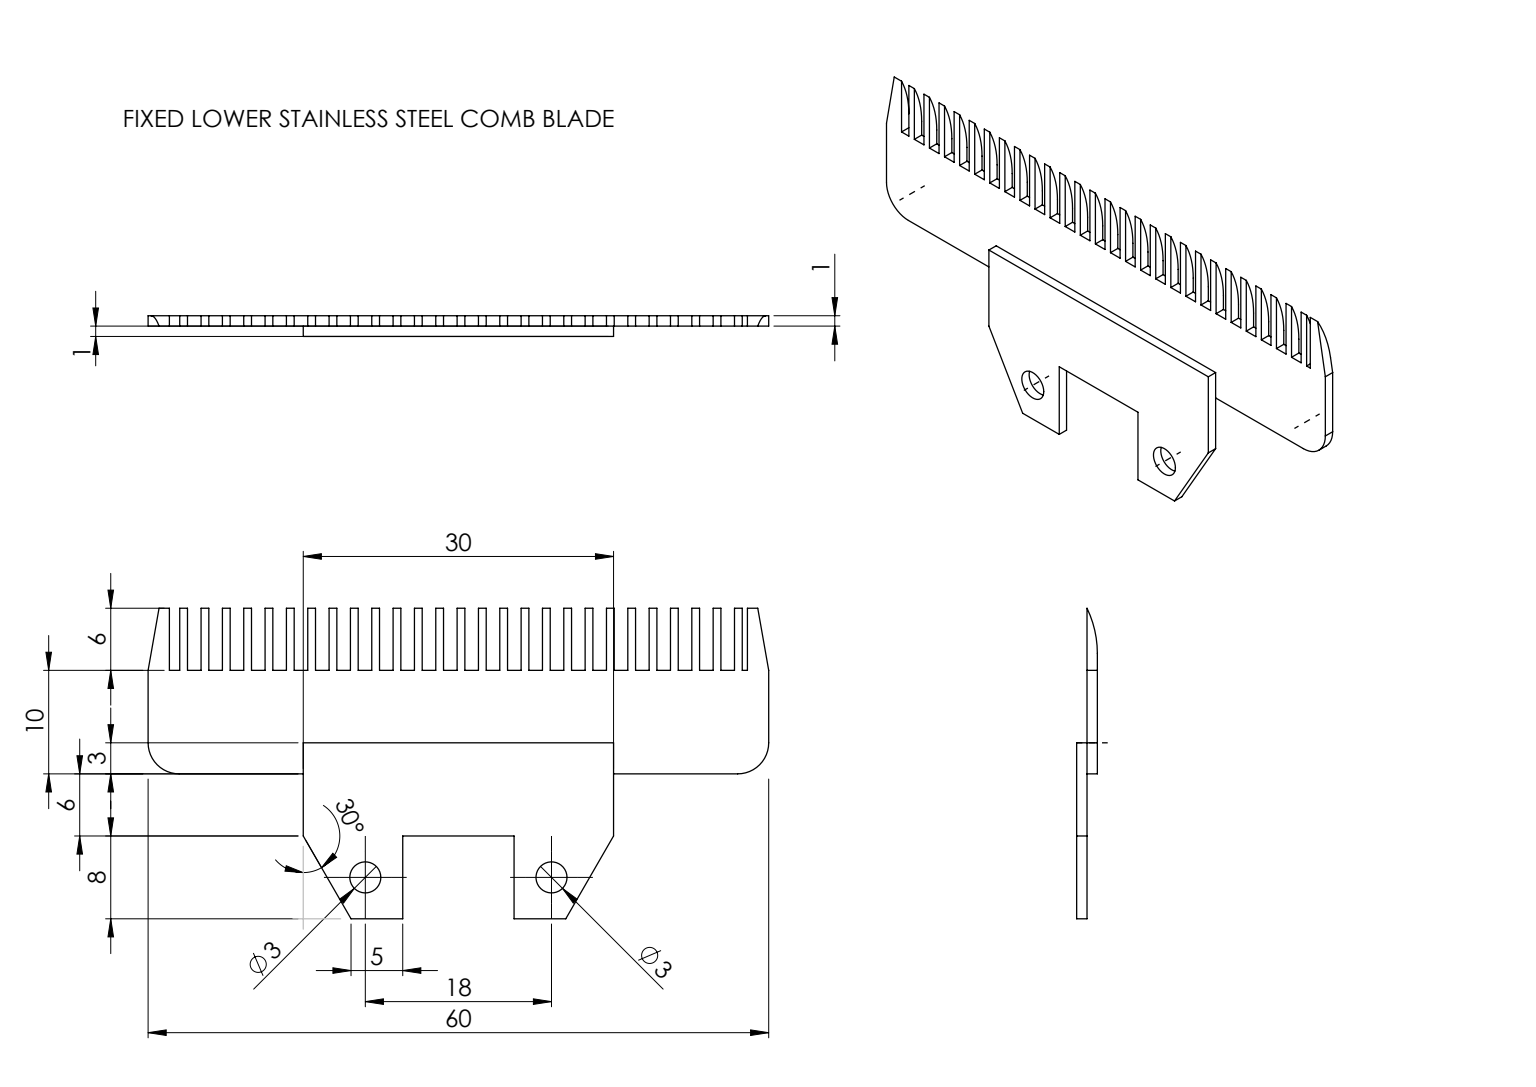
ISO-10303-21;
HEADER;
FILE_DESCRIPTION (('STEP AP214'),
    '1' );
FILE_NAME ('Fixed Lower Stainless Steel Comb Blade.step',
    '2026-10-04T16:38:04',
    ( '' ),
    ( '' ),
    'SwSTEP 2.0',
    'SolidWorks 2026',
    '' );
FILE_SCHEMA (( 'AUTOMOTIVE_DESIGN' ));
ENDSEC;

DATA;
#1=EDGE_CURVE ( 'NONE', #8973, #13899, #6324, .T. ) ;
#2=DIRECTION ( 'NONE',  ( -1.000000000000000000, 0.000000000000000000, 0.000000000000000000 ) ) ;
#6=AXIS2_PLACEMENT_3D ( 'NONE', #19220, #15754, #1437 ) ;
#8=CARTESIAN_POINT ( 'NONE',  ( -22.81633994409548549, 11.64110105645932691, 0.000000000000000000 ) ) ;
#13=VERTEX_POINT ( 'NONE', #12698 ) ;
#20=CARTESIAN_POINT ( 'NONE',  ( 29.44326362367961636, 13.15740888934567288, -2.785412301099487325E-16 ) ) ;
#23=CIRCLE ( 'NONE', #12706, 10.00000000000000000 ) ;
#24=DIRECTION ( 'NONE',  ( 1.000000000000000000, 0.000000000000000000, 0.000000000000000000 ) ) ;
#27=EDGE_CURVE ( 'NONE', #6657, #12771, #12900, .T. ) ;
#31=CARTESIAN_POINT ( 'NONE',  ( -18.69064177244175795, 11.64110105645932691, 0.000000000000000000 ) ) ;
#36=ADVANCED_FACE ( 'NONE', ( #7996 ), #7800, .T. ) ;
#38=CARTESIAN_POINT ( 'NONE',  ( 0.000000000000000000, 10.00000000000000000, 1.000000000000000000 ) ) ;
#39=CIRCLE ( 'NONE', #18741, 9.999999999999998224 ) ;
#43=VECTOR ( 'NONE', #1167, 1000.000000000000000 ) ;
#50=PLANE ( 'NONE',  #13438 ) ;
#51=PLANE ( 'NONE',  #17586 ) ;
#52=DIRECTION ( 'NONE',  ( 0.000000000000000000, 0.000000000000000000, 1.000000000000000000 ) ) ;
#62=DIRECTION ( 'NONE',  ( -5.782411586589356653E-16, 1.000000000000000000, 0.000000000000000000 ) ) ;
#73=AXIS2_PLACEMENT_3D ( 'NONE', #7626, #20402, #7929 ) ;
#74=DIRECTION ( 'NONE',  ( 1.000000000000000000, 0.000000000000000000, -0.000000000000000000 ) ) ;
#80=DIRECTION ( 'NONE',  ( -0.000000000000000000, -0.000000000000000000, -1.000000000000000000 ) ) ;
#81=EDGE_CURVE ( 'NONE', #12312, #20463, #4960, .T. ) ;
#93=DIRECTION ( 'NONE',  ( -0.000000000000000000, -0.000000000000000000, -1.000000000000000000 ) ) ;
#100=DIRECTION ( 'NONE',  ( 0.000000000000000000, 1.000000000000000000, 0.000000000000000000 ) ) ;
#104=ORIENTED_EDGE ( 'NONE', *, *, #13146, .F. ) ;
#118=EDGE_CURVE ( 'NONE', #8944, #9004, #361, .T. ) ;
#124=CARTESIAN_POINT ( 'NONE',  ( 27.94203811574920948, 16.00000000000000000, 1.000000000000000000 ) ) ;
#127=EDGE_LOOP ( 'NONE', ( #2197, #15477, #13303, #7881 ) ) ;
#129=CARTESIAN_POINT ( 'NONE',  ( 0.000000000000000000, 11.64110105645932691, 10.00000000000000000 ) ) ;
#130=FACE_OUTER_BOUND ( 'NONE', #18306, .T. ) ;
#131=APPLICATION_CONTEXT ( 'automotive_design' ) ;
#136=DIRECTION ( 'NONE',  ( 0.000000000000000000, 0.000000000000000000, -1.000000000000000000 ) ) ;
#140=ORIENTED_EDGE ( 'NONE', *, *, #2638, .T. ) ;
#142=CARTESIAN_POINT ( 'NONE',  ( 6.063547257480584207, 10.00000000000000000, 1.000000000000000000 ) ) ;
#145=EDGE_LOOP ( 'NONE', ( #572, #13357 ) ) ;
#149=EDGE_LOOP ( 'NONE', ( #17432, #19814, #17504, #3948 ) ) ;
#151=ORIENTED_EDGE ( 'NONE', *, *, #14900, .F. ) ;
#152=CARTESIAN_POINT ( 'NONE',  ( -27.94203811574921659, 9.999999999999998224, 1.000000000000000000 ) ) ;
#157=CARTESIAN_POINT ( 'NONE',  ( 0.000000000000000000, 10.00000000000000000, 1.000000000000000000 ) ) ;
#160=CARTESIAN_POINT ( 'NONE',  ( 27.00000000000000000, 3.000000000000000000, 1.000000000000000000 ) ) ;
#162=DIRECTION ( 'NONE',  ( -0.000000000000000000, -0.000000000000000000, -1.000000000000000000 ) ) ;
#171=ORIENTED_EDGE ( 'NONE', *, *, #6216, .T. ) ;
#172=ORIENTED_EDGE ( 'NONE', *, *, #1116, .F. ) ;
#173=DIRECTION ( 'NONE',  ( -0.000000000000000000, -0.000000000000000000, -1.000000000000000000 ) ) ;
#175=VERTEX_POINT ( 'NONE', #3806 ) ;
#176=CARTESIAN_POINT ( 'NONE',  ( -15.00000000000000000, 3.000000000000000000, 1.000000000000000000 ) ) ;
#184=EDGE_CURVE ( 'NONE', #2924, #1770, #13210, .T. ) ;
#193=VERTEX_POINT ( 'NONE', #561 ) ;
#194=FACE_OUTER_BOUND ( 'NONE', #14246, .T. ) ;
#196=LINE ( 'NONE', #13157, #16335 ) ;
#197=EDGE_CURVE ( 'NONE', #4053, #10774, #19608, .T. ) ;
#201=CARTESIAN_POINT ( 'NONE',  ( -8.376396343307449754, 11.64110105645932691, 0.000000000000000000 ) ) ;
#204=DIRECTION ( 'NONE',  ( 0.000000000000000000, -1.000000000000000000, 0.000000000000000000 ) ) ;
#219=CYLINDRICAL_SURFACE ( 'NONE', #18842, 10.00000000000000000 ) ;
#221=ORIENTED_EDGE ( 'NONE', *, *, #17663, .T. ) ;
#222=CARTESIAN_POINT ( 'NONE',  ( -14.56494360078803396, 0.000000000000000000, 0.000000000000000000 ) ) ;
#223=CYLINDRICAL_SURFACE ( 'NONE', #8699, 10.00000000000000000 ) ;
#226=CARTESIAN_POINT ( 'NONE',  ( 0.000000000000000000, 11.64110105645932691, 10.00000000000000000 ) ) ;
#227=EDGE_CURVE ( 'NONE', #2917, #11113, #5373, .T. ) ;
#234=EDGE_LOOP ( 'NONE', ( #6120, #13458, #16622, #14444 ) ) ;
#235=VECTOR ( 'NONE', #10575, 1000.000000000000000 ) ;
#240=EDGE_LOOP ( 'NONE', ( #2876, #19889, #3545, #20179 ) ) ;
#243=CARTESIAN_POINT ( 'NONE',  ( -0.000000000000000000, 10.00000000000000000, 0.000000000000000000 ) ) ;
#245=ORIENTED_EDGE ( 'NONE', *, *, #7610, .F. ) ;
#246=LINE ( 'NONE', #152, #17116 ) ;
#251=CARTESIAN_POINT ( 'NONE',  ( -7.500000000000000888, -9.999999999999992895, 1.000000000000000000 ) ) ;
#252=VECTOR ( 'NONE', #1364, 1000.000000000000000 ) ;
#256=LINE ( 'NONE', #3402, #19673 ) ;
#264=ADVANCED_FACE ( 'NONE', ( #16459 ), #18242, .T. ) ;
#269=CARTESIAN_POINT ( 'NONE',  ( -0.000000000000000000, 11.64110105645932691, 0.000000000000000000 ) ) ;
#271=ORIENTED_EDGE ( 'NONE', *, *, #10983, .T. ) ;
#273=VECTOR ( 'NONE', #18703, 1000.000000000000000 ) ;
#276=DIRECTION ( 'NONE',  ( 0.000000000000000000, 0.000000000000000000, 1.000000000000000000 ) ) ;
#280=AXIS2_PLACEMENT_3D ( 'NONE', #10758, #15558, #17129 ) ;
#283=FILL_AREA_STYLE ('',( #16193 ) ) ;
#285=DIRECTION ( 'NONE',  ( 1.000000000000000000, 0.000000000000000000, -0.000000000000000000 ) ) ;
#287=ORIENTED_EDGE ( 'NONE', *, *, #9934, .F. ) ;
#289=ADVANCED_FACE ( 'NONE', ( #9873 ), #19713, .T. ) ;
#298=CIRCLE ( 'NONE', #11982, 10.00000000000000000 ) ;
#301=EDGE_CURVE ( 'NONE', #14522, #1368, #8723, .T. ) ;
#309=CARTESIAN_POINT ( 'NONE',  ( 18.44064177244175440, 16.00000000000000000, 1.000000000000000000 ) ) ;
#310=EDGE_CURVE ( 'NONE', #175, #19704, #17077, .T. ) ;
#314=CIRCLE ( 'NONE', #14674, 10.00000000000000000 ) ;
#319=VECTOR ( 'NONE', #10177, 1000.000000000000000 ) ;
#320=DIRECTION ( 'NONE',  ( 0.000000000000000000, -0.000000000000000000, 1.000000000000000000 ) ) ;
#327=DIRECTION ( 'NONE',  ( 0.000000000000000000, 0.000000000000000000, -1.000000000000000000 ) ) ;
#330=EDGE_CURVE ( 'NONE', #20408, #13997, #13927, .T. ) ;
#333=CARTESIAN_POINT ( 'NONE',  ( -2.187849085826861550, 10.00000000000000000, 0.000000000000000000 ) ) ;
#336=CARTESIAN_POINT ( 'NONE',  ( 4.750698171653723989, 10.00000000000000000, 1.000000000000000000 ) ) ;
#338=EDGE_CURVE ( 'NONE', #6318, #18399, #16985, .T. ) ;
#343=PLANE ( 'NONE',  #7411 ) ;
#346=VERTEX_POINT ( 'NONE', #16765 ) ;
#348=CARTESIAN_POINT ( 'NONE',  ( -1.734723475976795735E-14, 10.00000000000004619, 1.000000000000000000 ) ) ;
#351=VERTEX_POINT ( 'NONE', #5579 ) ;
#356=EDGE_CURVE ( 'NONE', #19341, #13538, #2755, .T. ) ;
#359=DIRECTION ( 'NONE',  ( -5.782411586589356653E-16, 1.000000000000000000, 0.000000000000000000 ) ) ;
#361=LINE ( 'NONE', #7053, #18342 ) ;
#363=CARTESIAN_POINT ( 'NONE',  ( 0.000000000000000000, 10.00000000000000000, 1.000000000000000000 ) ) ;
#368=VECTOR ( 'NONE', #17912, 1000.000000000000000 ) ;
#378=VERTEX_POINT ( 'NONE', #17178 ) ;
#384=LINE ( 'NONE', #6768, #18444 ) ;
#388=ORIENTED_EDGE ( 'NONE', *, *, #15625, .T. ) ;
#392=DIRECTION ( 'NONE',  ( 0.000000000000000000, 0.000000000000000000, 1.000000000000000000 ) ) ;
#394=PRESENTATION_STYLE_ASSIGNMENT (( #14290 ) ) ;
#396=LINE ( 'NONE', #10120, #18568 ) ;
#405=CARTESIAN_POINT ( 'NONE',  ( 26.69203811574920238, 11.64110105645932691, 0.000000000000000000 ) ) ;
#409=EDGE_CURVE ( 'NONE', #6506, #12491, #9133, .T. ) ;
#411=VERTEX_POINT ( 'NONE', #5686 ) ;
#412=CARTESIAN_POINT ( 'NONE',  ( -27.94203811574921303, 11.64110105645932691, 10.00000000000000000 ) ) ;
#425=FACE_OUTER_BOUND ( 'NONE', #12281, .T. ) ;
#434=DIRECTION ( 'NONE',  ( -0.000000000000000000, -0.000000000000000000, -1.000000000000000000 ) ) ;
#440=DIRECTION ( 'NONE',  ( 1.000000000000000000, 0.000000000000000000, 0.000000000000000000 ) ) ;
#442=VECTOR ( 'NONE', #9719, 1000.000000000000000 ) ;
#446=CYLINDRICAL_SURFACE ( 'NONE', #17752, 10.00000000000000000 ) ;
#454=ORIENTED_EDGE ( 'NONE', *, *, #14597, .T. ) ;
#461=ADVANCED_FACE ( 'NONE', ( #3622 ), #6973, .T. ) ;
#466=DIRECTION ( 'NONE',  ( -0.000000000000000000, -0.000000000000000000, -1.000000000000000000 ) ) ;
#470=DIRECTION ( 'NONE',  ( 1.000000000000000000, 0.000000000000000000, 0.000000000000000000 ) ) ;
#489=DIRECTION ( 'NONE',  ( 0.000000000000000000, -1.000000000000000000, 0.000000000000000000 ) ) ;
#490=LINE ( 'NONE', #6775, #4650 ) ;
#501=ORIENTED_EDGE ( 'NONE', *, *, #15488, .T. ) ;
#503=CARTESIAN_POINT ( 'NONE',  ( 30.00000000000000000, 3.000000000000000000, 0.000000000000000000 ) ) ;
#508=VECTOR ( 'NONE', #11618, 1000.000000000000000 ) ;
#513=CARTESIAN_POINT ( 'NONE',  ( -0.000000000000000000, 11.64110105645932691, 0.000000000000000000 ) ) ;
#525=DIRECTION ( 'NONE',  ( 0.000000000000000000, 0.000000000000000000, -1.000000000000000000 ) ) ;
#527=ORIENTED_EDGE ( 'NONE', *, *, #9483, .F. ) ;
#531=FACE_OUTER_BOUND ( 'NONE', #8969, .T. ) ;
#532=ORIENTED_EDGE ( 'NONE', *, *, #6304, .F. ) ;
#534=LINE ( 'NONE', #6912, #4355 ) ;
#555=VECTOR ( 'NONE', #16159, 1000.000000000000000 ) ;
#556=CARTESIAN_POINT ( 'NONE',  ( 8.126396343307449754, 0.000000000000000000, 1.000000000000000000 ) ) ;
#561=CARTESIAN_POINT ( 'NONE',  ( 13.00209451496117374, 11.64110105645932691, 0.000000000000000000 ) ) ;
#562=CYLINDRICAL_SURFACE ( 'NONE', #14318, 10.00000000000000000 ) ;
#567=LINE ( 'NONE', #16465, #6029 ) ;
#572=ORIENTED_EDGE ( 'NONE', *, *, #19968, .T. ) ;
#574=LINE ( 'NONE', #19934, #13378 ) ;
#576=ORIENTED_EDGE ( 'NONE', *, *, #19487, .F. ) ;
#583=CARTESIAN_POINT ( 'NONE',  ( -3.500698171653725765, 11.64110105645932691, 0.000000000000000000 ) ) ;
#586=DIRECTION ( 'NONE',  ( 0.000000000000000000, 1.000000000000000000, -0.000000000000000000 ) ) ;
#587=PLANE ( 'NONE',  #2307 ) ;
#588=LINE ( 'NONE', #19745, #15656 ) ;
#594=EDGE_CURVE ( 'NONE', #13481, #20714, #588, .T. ) ;
#604=LINE ( 'NONE', #15142, #17681 ) ;
#606=SHAPE_DEFINITION_REPRESENTATION ( #14520, #19662 ) ;
#615=CARTESIAN_POINT ( 'NONE',  ( -8.376396343307449754, 11.64110105645932691, 10.00000000000000000 ) ) ;
#616=LINE ( 'NONE', #726, #14849 ) ;
#624=VECTOR ( 'NONE', #19202, 1000.000000000000000 ) ;
#629=ORIENTED_EDGE ( 'NONE', *, *, #10847, .F. ) ;
#630=ORIENTED_EDGE ( 'NONE', *, *, #4807, .F. ) ;
#634=CARTESIAN_POINT ( 'NONE',  ( 4.000698171653723101, 10.00000000000000000, 1.000000000000000000 ) ) ;
#636=LINE ( 'NONE', #7026, #13982 ) ;
#639=AXIS2_PLACEMENT_3D ( 'NONE', #157, #12701, #9776 ) ;
#655=ORIENTED_EDGE ( 'NONE', *, *, #12607, .T. ) ;
#658=DIRECTION ( 'NONE',  ( -1.000000000000000000, 0.000000000000000000, 0.000000000000000000 ) ) ;
#659=AXIS2_PLACEMENT_3D ( 'NONE', #17311, #5726, #12097 ) ;
#660=VECTOR ( 'NONE', #4913, 1000.000000000000000 ) ;
#662=DIRECTION ( 'NONE',  ( 1.000000000000000000, 0.000000000000000000, 0.000000000000000000 ) ) ;
#663=CARTESIAN_POINT ( 'NONE',  ( -26.94203811574920593, 0.000000000000000000, 0.000000000000000000 ) ) ;
#665=DIRECTION ( 'NONE',  ( 1.000000000000000000, 0.000000000000000000, -0.000000000000000000 ) ) ;
#667=DIRECTION ( 'NONE',  ( 1.000000000000000000, 0.000000000000000000, -0.000000000000000000 ) ) ;
#669=EDGE_CURVE ( 'NONE', #13945, #9626, #15323, .T. ) ;
#676=ORIENTED_EDGE ( 'NONE', *, *, #19705, .T. ) ;
#680=CIRCLE ( 'NONE', #7376, 10.00000000000000000 ) ;
#682=VERTEX_POINT ( 'NONE', #12399 ) ;
#687=LINE ( 'NONE', #13638, #17158 ) ;
#690=EDGE_CURVE ( 'NONE', #11466, #16861, #9064, .T. ) ;
#691=AXIS2_PLACEMENT_3D ( 'NONE', #3479, #1908, #9120 ) ;
#696=VECTOR ( 'NONE', #19733, 1000.000000000000000 ) ;
#710=ORIENTED_EDGE ( 'NONE', *, *, #2316, .F. ) ;
#711=AXIS2_PLACEMENT_3D ( 'NONE', #20236, #7367, #5796 ) ;
#712=CARTESIAN_POINT ( 'NONE',  ( 22.56633994409548194, 16.00000000000000000, 1.000000000000000000 ) ) ;
#717=ORIENTED_EDGE ( 'NONE', *, *, #19240, .F. ) ;
#718=EDGE_CURVE ( 'NONE', #4809, #5545, #7592, .T. ) ;
#719=FACE_OUTER_BOUND ( 'NONE', #15342, .T. ) ;
#725=DIRECTION ( 'NONE',  ( -0.000000000000000000, 0.000000000000000000, -1.000000000000000000 ) ) ;
#726=CARTESIAN_POINT ( 'NONE',  ( -20.75349085826862350, 10.00000000000000000, 1.000000000000000000 ) ) ;
#727=VECTOR ( 'NONE', #14197, 1000.000000000000000 ) ;
#743=DIRECTION ( 'NONE',  ( 0.000000000000000000, 0.000000000000000000, 1.000000000000000000 ) ) ;
#748=DIRECTION ( 'NONE',  ( 0.000000000000000000, 0.000000000000000000, -1.000000000000000000 ) ) ;
#766=FACE_OUTER_BOUND ( 'NONE', #18789, .T. ) ;
#767=ORIENTED_EDGE ( 'NONE', *, *, #8340, .T. ) ;
#771=CARTESIAN_POINT ( 'NONE',  ( 16.37779268661489596, 0.000000000000000000, 1.000000000000000000 ) ) ;
#772=DIRECTION ( 'NONE',  ( 0.000000000000000000, -0.000000000000000000, -1.000000000000000000 ) ) ;
#773=CARTESIAN_POINT ( 'NONE',  ( 20.50349085826861995, 0.000000000000000000, 0.000000000000000000 ) ) ;
#777=DIRECTION ( 'NONE',  ( 1.000000000000000000, 0.000000000000000000, 0.000000000000000000 ) ) ;
#784=EDGE_CURVE ( 'NONE', #4291, #411, #2676, .T. ) ;
#789=CARTESIAN_POINT ( 'NONE',  ( -27.94203811574922725, 3.231447299068595019E-14, 1.000000000000000000 ) ) ;
#793=ORIENTED_EDGE ( 'NONE', *, *, #7303, .T. ) ;
#797=VECTOR ( 'NONE', #17296, 1000.000000000000000 ) ;
#798=ORIENTED_EDGE ( 'NONE', *, *, #5836, .F. ) ;
#805=CARTESIAN_POINT ( 'NONE',  ( -18.69064177244175795, 11.64110105645932691, 10.00000000000000000 ) ) ;
#815=LINE ( 'NONE', #7299, #19326 ) ;
#823=LINE ( 'NONE', #10649, #7633 ) ;
#832=ORIENTED_EDGE ( 'NONE', *, *, #2086, .F. ) ;
#833=ADVANCED_FACE ( 'NONE', ( #17106 ), #10937, .T. ) ;
#835=DIRECTION ( 'NONE',  ( 1.000000000000000000, -0.000000000000000000, 0.000000000000000000 ) ) ;
#839=ORIENTED_EDGE ( 'NONE', *, *, #13617, .T. ) ;
#850=CARTESIAN_POINT ( 'NONE',  ( -2.187849085826861550, 10.00000000000000000, 1.000000000000000000 ) ) ;
#855=AXIS2_PLACEMENT_3D ( 'NONE', #14509, #8242, #12934 ) ;
#856=CARTESIAN_POINT ( 'NONE',  ( -0.000000000000000000, 10.00000000000000000, 0.000000000000000000 ) ) ;
#873=DIRECTION ( 'NONE',  ( 1.000000000000000000, 0.000000000000000000, 0.000000000000000000 ) ) ;
#876=CARTESIAN_POINT ( 'NONE',  ( 20.50349085826861995, 0.000000000000000000, 1.000000000000000000 ) ) ;
#886=VERTEX_POINT ( 'NONE', #6224 ) ;
#888=LINE ( 'NONE', #10512, #20085 ) ;
#897=ADVANCED_FACE ( 'NONE', ( #7803 ), #12901, .T. ) ;
#900=DIRECTION ( 'NONE',  ( 0.000000000000000000, -0.000000000000000000, 1.000000000000000000 ) ) ;
#903=CARTESIAN_POINT ( 'NONE',  ( 8.126396343307449754, 11.64110105645932691, 0.000000000000000000 ) ) ;
#913=FACE_OUTER_BOUND ( 'NONE', #2688, .T. ) ;
#920=ADVANCED_FACE ( 'NONE', ( #1618 ), #9469, .T. ) ;
#932=VERTEX_POINT ( 'NONE', #17729 ) ;
#939=EDGE_LOOP ( 'NONE', ( #171, #11278, #1339, #9867 ) ) ;
#949=EDGE_CURVE ( 'NONE', #20101, #8920, #1728, .T. ) ;
#952=CARTESIAN_POINT ( 'NONE',  ( 27.94203811574922725, 3.231447299068595019E-14, 0.000000000000000000 ) ) ;
#962=VERTEX_POINT ( 'NONE', #11238 ) ;
#964=CARTESIAN_POINT ( 'NONE',  ( 4.750698171653723989, 16.00000000000000000, 1.000000000000000000 ) ) ;
#965=VERTEX_POINT ( 'NONE', #20572 ) ;
#966=ORIENTED_EDGE ( 'NONE', *, *, #1652, .F. ) ;
#972=EDGE_CURVE ( 'NONE', #9402, #17667, #9669, .T. ) ;
#976=CARTESIAN_POINT ( 'NONE',  ( 10.18924542913430820, 10.00000000000000000, 1.000000000000000000 ) ) ;
#978=DIRECTION ( 'NONE',  ( 0.000000000000000000, 1.000000000000000000, 0.000000000000000000 ) ) ;
#986=CARTESIAN_POINT ( 'NONE',  ( -1.437849085826860884, 11.64110105645932691, 0.000000000000000000 ) ) ;
#991=ORIENTED_EDGE ( 'NONE', *, *, #5535, .F. ) ;
#994=ORIENTED_EDGE ( 'NONE', *, *, #11563, .T. ) ;
#996=LINE ( 'NONE', #20151, #19846 ) ;
#1000=CARTESIAN_POINT ( 'NONE',  ( 25.37918902992234393, 0.000000000000000000, 1.000000000000000000 ) ) ;
#1001=LINE ( 'NONE', #7082, #16680 ) ;
#1002=( GEOMETRIC_REPRESENTATION_CONTEXT ( 3 ) GLOBAL_UNCERTAINTY_ASSIGNED_CONTEXT ( ( #2948 ) ) GLOBAL_UNIT_ASSIGNED_CONTEXT ( ( #5234, #16426, #16621 ) ) REPRESENTATION_CONTEXT ( 'NONE', 'WORKASPACE' ) );
#1003=CARTESIAN_POINT ( 'NONE',  ( 23.31633994409548549, 0.000000000000000000, 1.000000000000000000 ) ) ;
#1006=AXIS2_PLACEMENT_3D ( 'NONE', #15854, #3208, #9485 ) ;
#1007=VECTOR ( 'NONE', #12119, 1000.000000000000000 ) ;
#1015=ADVANCED_FACE ( 'NONE', ( #8213 ), #4758, .T. ) ;
#1017=EDGE_LOOP ( 'NONE', ( #9052, #2300, #4060, #7390 ) ) ;
#1022=ORIENTED_EDGE ( 'NONE', *, *, #10245, .T. ) ;
#1023=CARTESIAN_POINT ( 'NONE',  ( -15.00000000000000000, -6.000000000000000000, 2.000000000000000000 ) ) ;
#1024=FACE_OUTER_BOUND ( 'NONE', #15421, .T. ) ;
#1031=ORIENTED_EDGE ( 'NONE', *, *, #1736, .T. ) ;
#1032=DIRECTION ( 'NONE',  ( 1.000000000000000000, 0.000000000000000000, -0.000000000000000000 ) ) ;
#1033=CARTESIAN_POINT ( 'NONE',  ( -0.000000000000000000, 10.00000000000000000, 0.000000000000000000 ) ) ;
#1042=VECTOR ( 'NONE', #2570, 1000.000000000000000 ) ;
#1043=AXIS2_PLACEMENT_3D ( 'NONE', #17057, #2736, #9115 ) ;
#1046=CARTESIAN_POINT ( 'NONE',  ( -5.381197846483055436, -14.00000000000000000, 2.000000000000000000 ) ) ;
#1060=EDGE_CURVE ( 'NONE', #11555, #13250, #3497, .T. ) ;
#1062=CARTESIAN_POINT ( 'NONE',  ( 18.44064177244175440, 10.00000000000000000, 1.000000000000000000 ) ) ;
#1063=VECTOR ( 'NONE', #10481, 1000.000000000000000 ) ;
#1064=CARTESIAN_POINT ( 'NONE',  ( -16.62779268661489951, 11.64110105645932691, 10.00000000000000000 ) ) ;
#1073=AXIS2_PLACEMENT_3D ( 'NONE', #16519, #16419, #13270 ) ;
#1079=CARTESIAN_POINT ( 'NONE',  ( -0.000000000000000000, 11.64110105645932691, 0.000000000000000000 ) ) ;
#1085=DIRECTION ( 'NONE',  ( 0.000000000000000000, 1.000000000000000000, -0.000000000000000000 ) ) ;
#1087=ADVANCED_FACE ( 'NONE', ( #2230 ), #18348, .T. ) ;
#1089=DIRECTION ( 'NONE',  ( -1.000000000000000000, 0.000000000000000000, 0.000000000000000000 ) ) ;
#1091=DIRECTION ( 'NONE',  ( 0.000000000000000000, 0.000000000000000000, 1.000000000000000000 ) ) ;
#1099=EDGE_CURVE ( 'NONE', #2580, #20101, #18033, .T. ) ;
#1102=ORIENTED_EDGE ( 'NONE', *, *, #4112, .T. ) ;
#1103=ADVANCED_FACE ( 'NONE', ( #10185 ), #2134, .T. ) ;
#1108=VECTOR ( 'NONE', #14446, 1000.000000000000000 ) ;
#1116=EDGE_CURVE ( 'NONE', #2917, #8843, #13323, .T. ) ;
#1121=CARTESIAN_POINT ( 'NONE',  ( -0.000000000000000000, 10.00000000000000000, 0.000000000000000000 ) ) ;
#1123=CARTESIAN_POINT ( 'NONE',  ( -30.80549002841696193, 5.431839045955507927, 1.000000000000000000 ) ) ;
#1130=EDGE_LOOP ( 'NONE', ( #10669, #9207, #839, #8430 ) ) ;
#1133=ORIENTED_EDGE ( 'NONE', *, *, #10725, .T. ) ;
#1138=CARTESIAN_POINT ( 'NONE',  ( 18.44064177244175440, 0.000000000000000000, 1.000000000000000000 ) ) ;
#1139=EDGE_CURVE ( 'NONE', #18061, #13178, #5166, .T. ) ;
#1140=LINE ( 'NONE', #1033, #20003 ) ;
#1143=LINE ( 'NONE', #10551, #6290 ) ;
#1144=CARTESIAN_POINT ( 'NONE',  ( 25.37918902992234393, 10.00000000000000000, 0.000000000000000000 ) ) ;
#1156=ORIENTED_EDGE ( 'NONE', *, *, #3778, .T. ) ;
#1167=DIRECTION ( 'NONE',  ( 1.156482317317871133E-15, -1.000000000000000000, 0.000000000000000000 ) ) ;
#1169=LINE ( 'NONE', #856, #1063 ) ;
#1172=EDGE_CURVE ( 'NONE', #20035, #2663, #3906, .T. ) ;
#1174=EDGE_CURVE ( 'NONE', #8843, #4699, #14987, .T. ) ;
#1179=FACE_OUTER_BOUND ( 'NONE', #10750, .T. ) ;
#1185=VECTOR ( 'NONE', #17236, 1000.000000000000000 ) ;
#1188=DIRECTION ( 'NONE',  ( 0.000000000000000000, 0.000000000000000000, 1.000000000000000000 ) ) ;
#1190=PLANE ( 'NONE',  #11495 ) ;
#1197=ADVANCED_FACE ( 'NONE', ( #5478 ), #562, .T. ) ;
#1200=APPLICATION_CONTEXT ( 'automotive_design' ) ;
#1207=EDGE_CURVE ( 'NONE', #1851, #19958, #13522, .T. ) ;
#1210=EDGE_LOOP ( 'NONE', ( #3460, #4701, #11385, #3949 ) ) ;
#1215=LINE ( 'NONE', #19203, #3009 ) ;
#1230=CARTESIAN_POINT ( 'NONE',  ( -15.00000000000000000, -6.000000000000000000, 2.000000000000000000 ) ) ;
#1235=VECTOR ( 'NONE', #15090, 1000.000000000000000 ) ;
#1238=CARTESIAN_POINT ( 'NONE',  ( -10.43924542913431175, 0.000000000000000000, 1.000000000000000000 ) ) ;
#1239=EDGE_CURVE ( 'NONE', #19704, #9634, #8725, .T. ) ;
#1240=ADVANCED_FACE ( 'NONE', ( #11951 ), #5996, .T. ) ;
#1242=CARTESIAN_POINT ( 'NONE',  ( -24.12918902992234393, 10.00000000000000000, 0.000000000000000000 ) ) ;
#1249=ORIENTED_EDGE ( 'NONE', *, *, #3446, .F. ) ;
#1261=ORIENTED_EDGE ( 'NONE', *, *, #17407, .T. ) ;
#1262=DIRECTION ( 'NONE',  ( -0.000000000000000000, 0.000000000000000000, -1.000000000000000000 ) ) ;
#1268=FACE_OUTER_BOUND ( 'NONE', #18251, .T. ) ;
#1280=VECTOR ( 'NONE', #19650, 1000.000000000000000 ) ;
#1281=EDGE_CURVE ( 'NONE', #3253, #12082, #13929, .T. ) ;
#1283=VERTEX_POINT ( 'NONE', #976 ) ;
#1289=CARTESIAN_POINT ( 'NONE',  ( -7.626396343307448866, 0.000000000000000000, 1.000000000000000000 ) ) ;
#1291=VECTOR ( 'NONE', #2912, 1000.000000000000000 ) ;
#1295=ORIENTED_EDGE ( 'NONE', *, *, #5909, .F. ) ;
#1297=DIRECTION ( 'NONE',  ( -0.000000000000000000, -0.000000000000000000, -1.000000000000000000 ) ) ;
#1304=ORIENTED_EDGE ( 'NONE', *, *, #16771, .F. ) ;
#1305=VECTOR ( 'NONE', #15964, 1000.000000000000000 ) ;
#1306=ORIENTED_EDGE ( 'NONE', *, *, #3962, .F. ) ;
#1312=CARTESIAN_POINT ( 'NONE',  ( 1.937849085826861328, 0.000000000000000000, 1.000000000000000000 ) ) ;
#1313=EDGE_CURVE ( 'NONE', #19341, #3875, #3984, .T. ) ;
#1314=EDGE_CURVE ( 'NONE', #18960, #13229, #314, .T. ) ;
#1317=CARTESIAN_POINT ( 'NONE',  ( 4.000698171653723101, 10.00000000000000000, 0.000000000000000000 ) ) ;
#1321=DIRECTION ( 'NONE',  ( 1.000000000000000000, 0.000000000000000000, 0.000000000000000000 ) ) ;
#1322=VECTOR ( 'NONE', #11570, 1000.000000000000000 ) ;
#1323=DIRECTION ( 'NONE',  ( 0.000000000000000000, 0.000000000000000000, 1.000000000000000000 ) ) ;
#1325=CARTESIAN_POINT ( 'NONE',  ( 21.25349085826861995, 10.00000000000000000, 1.000000000000000000 ) ) ;
#1335=DIRECTION ( 'NONE',  ( 1.000000000000000000, 0.000000000000000000, 0.000000000000000000 ) ) ;
#1337=CARTESIAN_POINT ( 'NONE',  ( -7.626396343307448866, 10.00000000000000000, 0.000000000000000000 ) ) ;
#1338=EDGE_CURVE ( 'NONE', #10660, #19958, #5662, .T. ) ;
#1339=ORIENTED_EDGE ( 'NONE', *, *, #3529, .F. ) ;
#1342=ORIENTED_EDGE ( 'NONE', *, *, #13749, .F. ) ;
#1351=DIRECTION ( 'NONE',  ( -0.000000000000000000, 0.000000000000000000, -1.000000000000000000 ) ) ;
#1357=ORIENTED_EDGE ( 'NONE', *, *, #81, .T. ) ;
#1364=DIRECTION ( 'NONE',  ( 1.000000000000000000, 0.000000000000000000, 0.000000000000000000 ) ) ;
#1365=ORIENTED_EDGE ( 'NONE', *, *, #8366, .F. ) ;
#1366=EDGE_CURVE ( 'NONE', #18502, #13489, #4431, .T. ) ;
#1368=VERTEX_POINT ( 'NONE', #16768 ) ;
#1384=ORIENTED_EDGE ( 'NONE', *, *, #2193, .F. ) ;
#1387=ORIENTED_EDGE ( 'NONE', *, *, #5301, .T. ) ;
#1389=ORIENTED_EDGE ( 'NONE', *, *, #4000, .T. ) ;
#1396=LINE ( 'NONE', #4624, #11203 ) ;
#1398=DIRECTION ( 'NONE',  ( 0.000000000000000000, -0.000000000000000000, 1.000000000000000000 ) ) ;
#1405=DIRECTION ( 'NONE',  ( 1.000000000000000000, 0.000000000000000000, -0.000000000000000000 ) ) ;
#1409=EDGE_CURVE ( 'NONE', #3062, #10193, #8830, .T. ) ;
#1416=VECTOR ( 'NONE', #15941, 1000.000000000000000 ) ;
#1419=CARTESIAN_POINT ( 'NONE',  ( 0.000000000000000000, 16.00000000000000000, 1.000000000000000000 ) ) ;
#1421=DIRECTION ( 'NONE',  ( 0.000000000000000000, -0.000000000000000000, 1.000000000000000000 ) ) ;
#1427=LINE ( 'NONE', #10849, #1700 ) ;
#1437=DIRECTION ( 'NONE',  ( 0.000000000000000000, 0.000000000000000000, 1.000000000000000000 ) ) ;
#1441=VERTEX_POINT ( 'NONE', #9034 ) ;
#1445=VECTOR ( 'NONE', #15787, 1000.000000000000000 ) ;
#1462=CARTESIAN_POINT ( 'NONE',  ( 10.18924542913430820, 11.64110105645932691, 0.000000000000000000 ) ) ;
#1465=LINE ( 'NONE', #20414, #442 ) ;
#1466=ORIENTED_EDGE ( 'NONE', *, *, #3446, .T. ) ;
#1468=CARTESIAN_POINT ( 'NONE',  ( -0.000000000000000000, 11.64110105645932691, 0.000000000000000000 ) ) ;
#1471=ADVANCED_FACE ( 'NONE', ( #17386 ), #19074, .F. ) ;
#1472=EDGE_CURVE ( 'NONE', #13772, #2830, #9444, .T. ) ;
#1473=CARTESIAN_POINT ( 'NONE',  ( -15.00000000000000000, -6.000000000000000000, 2.000000000000000000 ) ) ;
#1475=AXIS2_PLACEMENT_3D ( 'NONE', #10527, #20476, #6132 ) ;
#1493=EDGE_CURVE ( 'NONE', #378, #6312, #19762, .T. ) ;
#1500=ORIENTED_EDGE ( 'NONE', *, *, #3525, .F. ) ;
#1502=CARTESIAN_POINT ( 'NONE',  ( 2.687849085826861995, 11.64110105645932691, 10.00000000000000000 ) ) ;
#1512=CYLINDRICAL_SURFACE ( 'NONE', #10435, 1.499999999999996891 ) ;
#1517=DIRECTION ( 'NONE',  ( -0.000000000000000000, -0.000000000000000000, -1.000000000000000000 ) ) ;
#1518=DIRECTION ( 'NONE',  ( 0.000000000000000000, 1.000000000000000000, -0.000000000000000000 ) ) ;
#1520=LINE ( 'NONE', #19106, #4362 ) ;
#1533=FACE_OUTER_BOUND ( 'NONE', #19932, .T. ) ;
#1535=CARTESIAN_POINT ( 'NONE',  ( 15.06494360078803041, 10.00000000000000000, 1.000000000000000000 ) ) ;
#1536=ORIENTED_EDGE ( 'NONE', *, *, #15092, .T. ) ;
#1542=CARTESIAN_POINT ( 'NONE',  ( -28.94203811574919882, 16.00000000000000000, 1.000000000000000000 ) ) ;
#1547=CARTESIAN_POINT ( 'NONE',  ( -22.06633994409548194, 11.64110105645932691, 0.000000000000000000 ) ) ;
#1559=ORIENTED_EDGE ( 'NONE', *, *, #20383, .T. ) ;
#1563=ORIENTED_EDGE ( 'NONE', *, *, #16412, .F. ) ;
#1566=ADVANCED_FACE ( 'NONE', ( #17275 ), #12987, .F. ) ;
#1567=FACE_OUTER_BOUND ( 'NONE', #5065, .T. ) ;
#1569=VECTOR ( 'NONE', #6938, 1000.000000000000000 ) ;
#1584=EDGE_CURVE ( 'NONE', #16102, #14797, #3048, .T. ) ;
#1585=ORIENTED_EDGE ( 'NONE', *, *, #1860, .F. ) ;
#1587=CARTESIAN_POINT ( 'NONE',  ( 0.6250000000000005551, 11.64110105645932691, 10.00000000000000000 ) ) ;
#1590=DIRECTION ( 'NONE',  ( 0.000000000000000000, 0.000000000000000000, -1.000000000000000000 ) ) ;
#1598=ORIENTED_EDGE ( 'NONE', *, *, #17190, .F. ) ;
#1600=LINE ( 'NONE', #38, #14047 ) ;
#1608=VERTEX_POINT ( 'NONE', #14141 ) ;
#1609=EDGE_CURVE ( 'NONE', #10227, #14087, #6299, .T. ) ;
#1612=CARTESIAN_POINT ( 'NONE',  ( 10.38119784648305810, -14.00000000000000000, 1.000000000000000000 ) ) ;
#1614=VECTOR ( 'NONE', #5297, 1000.000000000000000 ) ;
#1615=VECTOR ( 'NONE', #2064, 1000.000000000000000 ) ;
#1618=FACE_OUTER_BOUND ( 'NONE', #16736, .T. ) ;
#1633=VERTEX_POINT ( 'NONE', #19689 ) ;
#1635=LINE ( 'NONE', #2801, #17559 ) ;
#1637=VECTOR ( 'NONE', #15038, 1000.000000000000000 ) ;
#1638=VERTEX_POINT ( 'NONE', #10165 ) ;
#1652=EDGE_CURVE ( 'NONE', #3666, #3062, #1902, .T. ) ;
#1658=FACE_OUTER_BOUND ( 'NONE', #18286, .T. ) ;
#1660=ORIENTED_EDGE ( 'NONE', *, *, #8284, .T. ) ;
#1672=CARTESIAN_POINT ( 'NONE',  ( -15.00000000000000000, 0.000000000000000000, 1.000000000000000000 ) ) ;
#1675=COLOUR_RGB ( '', 0.72549020, 0.75294118, 0.79215686) ;
#1676=LINE ( 'NONE', #6085, #15019 ) ;
#1682=EDGE_CURVE ( 'NONE', #18231, #20454, #4041, .T. ) ;
#1689=VERTEX_POINT ( 'NONE', #15071 ) ;
#1694=CARTESIAN_POINT ( 'NONE',  ( 24.62918902992234038, 10.00000000000000000, 1.000000000000000000 ) ) ;
#1699=DIRECTION ( 'NONE',  ( 1.000000000000000000, 0.000000000000000000, -0.000000000000000000 ) ) ;
#1700=VECTOR ( 'NONE', #16899, 1000.000000000000000 ) ;
#1703=CARTESIAN_POINT ( 'NONE',  ( 16.37779268661489596, 16.00000000000000000, 1.000000000000000000 ) ) ;
#1718=AXIS2_PLACEMENT_3D ( 'NONE', #11317, #19284, #6518 ) ;
#1722=EDGE_LOOP ( 'NONE', ( #20152, #4422, #12846, #17772 ) ) ;
#1723=ORIENTED_EDGE ( 'NONE', *, *, #4575, .F. ) ;
#1725=DIRECTION ( 'NONE',  ( 1.000000000000000000, 0.000000000000000000, 0.000000000000000000 ) ) ;
#1728=LINE ( 'NONE', #3193, #10664 ) ;
#1730=LINE ( 'NONE', #12597, #15873 ) ;
#1731=CARTESIAN_POINT ( 'NONE',  ( 0.000000000000000000, 10.00000000000000000, 1.000000000000000000 ) ) ;
#1733=DIRECTION ( 'NONE',  ( -0.000000000000000000, -0.000000000000000000, -1.000000000000000000 ) ) ;
#1734=LINE ( 'NONE', #14377, #15987 ) ;
#1736=EDGE_CURVE ( 'NONE', #11041, #2445, #5146, .T. ) ;
#1742=VERTEX_POINT ( 'NONE', #13398 ) ;
#1744=LINE ( 'NONE', #11252, #18740 ) ;
#1745=ORIENTED_EDGE ( 'NONE', *, *, #19077, .T. ) ;
#1747=VECTOR ( 'NONE', #1848, 1000.000000000000000 ) ;
#1749=ORIENTED_EDGE ( 'NONE', *, *, #17411, .T. ) ;
#1754=DIRECTION ( 'NONE',  ( 1.000000000000000000, 0.000000000000000000, 0.000000000000000000 ) ) ;
#1756=DIRECTION ( 'NONE',  ( 1.000000000000000000, 0.000000000000000000, 0.000000000000000000 ) ) ;
#1766=ORIENTED_EDGE ( 'NONE', *, *, #20416, .T. ) ;
#1767=LINE ( 'NONE', #8155, #14956 ) ;
#1770=VERTEX_POINT ( 'NONE', #14962 ) ;
#1772=EDGE_CURVE ( 'NONE', #4081, #14620, #2311, .T. ) ;
#1784=CIRCLE ( 'NONE', #2435, 10.00000000000000000 ) ;
#1789=ORIENTED_EDGE ( 'NONE', *, *, #16619, .T. ) ;
#1792=CARTESIAN_POINT ( 'NONE',  ( 0.000000000000000000, 11.64110105645932691, 10.00000000000000000 ) ) ;
#1793=CARTESIAN_POINT ( 'NONE',  ( 0.000000000000000000, 0.000000000000000000, 0.000000000000000000 ) ) ;
#1795=ORIENTED_EDGE ( 'NONE', *, *, #10684, .T. ) ;
#1801=DIRECTION ( 'NONE',  ( 1.000000000000000000, -0.000000000000000000, 0.000000000000000000 ) ) ;
#1807=LINE ( 'NONE', #6108, #14741 ) ;
#1810=ORIENTED_EDGE ( 'NONE', *, *, #17827, .F. ) ;
#1812=FACE_OUTER_BOUND ( 'NONE', #16104, .T. ) ;
#1819=ORIENTED_EDGE ( 'NONE', *, *, #6500, .T. ) ;
#1829=ADVANCED_FACE ( 'NONE', ( #1268 ), #3988, .T. ) ;
#1840=ORIENTED_EDGE ( 'NONE', *, *, #9665, .F. ) ;
#1848=DIRECTION ( 'NONE',  ( -1.000000000000000000, -1.156482317317871725E-16, -0.000000000000000000 ) ) ;
#1849=EDGE_CURVE ( 'NONE', #14060, #19940, #8808, .T. ) ;
#1851=VERTEX_POINT ( 'NONE', #4297 ) ;
#1853=CARTESIAN_POINT ( 'NONE',  ( -0.000000000000000000, 10.00000000000000000, 0.000000000000000000 ) ) ;
#1860=EDGE_CURVE ( 'NONE', #20119, #8195, #13809, .T. ) ;
#1868=DIRECTION ( 'NONE',  ( 1.000000000000000000, 0.000000000000000000, 0.000000000000000000 ) ) ;
#1872=EDGE_CURVE ( 'NONE', #4053, #6506, #19903, .T. ) ;
#1878=CYLINDRICAL_SURFACE ( 'NONE', #12140, 1.499999999999999556 ) ;
#1882=DIRECTION ( 'NONE',  ( 0.000000000000000000, 0.000000000000000000, 1.000000000000000000 ) ) ;
#1889=LINE ( 'NONE', #18105, #20451 ) ;
#1895=DIRECTION ( 'NONE',  ( 0.000000000000000000, 1.000000000000000000, -0.000000000000000000 ) ) ;
#1898=CARTESIAN_POINT ( 'NONE',  ( 24.62918902992234038, 11.64110105645932691, 10.00000000000000000 ) ) ;
#1902=LINE ( 'NONE', #16236, #16080 ) ;
#1905=CARTESIAN_POINT ( 'NONE',  ( 0.000000000000000000, 10.00000000000000000, 1.000000000000000000 ) ) ;
#1907=EDGE_CURVE ( 'NONE', #17851, #19480, #5772, .T. ) ;
#1908=DIRECTION ( 'NONE',  ( 1.000000000000000000, -0.000000000000000000, 0.000000000000000000 ) ) ;
#1922=DIRECTION ( 'NONE',  ( -1.000000000000000000, 0.000000000000000000, 0.000000000000000000 ) ) ;
#1927=CARTESIAN_POINT ( 'NONE',  ( -5.381197846483055436, -6.000000000000000000, 1.000000000000000000 ) ) ;
#1930=DIRECTION ( 'NONE',  ( 1.000000000000000000, 0.000000000000000000, 0.000000000000000000 ) ) ;
#1945=VECTOR ( 'NONE', #14818, 1000.000000000000000 ) ;
#1948=EDGE_CURVE ( 'NONE', #3754, #20490, #16945, .T. ) ;
#1962=EDGE_CURVE ( 'NONE', #8181, #14649, #15384, .T. ) ;
#1963=ORIENTED_EDGE ( 'NONE', *, *, #12166, .T. ) ;
#1967=ORIENTED_EDGE ( 'NONE', *, *, #10492, .T. ) ;
#1969=CARTESIAN_POINT ( 'NONE',  ( 0.000000000000000000, 16.00000000000000000, 1.000000000000000000 ) ) ;
#1970=EDGE_LOOP ( 'NONE', ( #4283, #1261, #13717, #9024 ) ) ;
#1976=ORIENTED_EDGE ( 'NONE', *, *, #18365, .F. ) ;
#1984=VECTOR ( 'NONE', #19824, 1000.000000000000000 ) ;
#1992=CARTESIAN_POINT ( 'NONE',  ( 23.31633994409548549, 10.00000000000000000, 1.000000000000000000 ) ) ;
#1999=ORIENTED_EDGE ( 'NONE', *, *, #17117, .T. ) ;
#2003=ADVANCED_FACE ( 'NONE', ( #10479 ), #2417, .T. ) ;
#2007=LINE ( 'NONE', #1419, #18889 ) ;
#2009=VECTOR ( 'NONE', #12857, 1000.000000000000000 ) ;
#2017=PLANE ( 'NONE',  #19417 ) ;
#2031=CARTESIAN_POINT ( 'NONE',  ( -26.19203811574920593, 0.000000000000000000, 1.000000000000000000 ) ) ;
#2044=EDGE_LOOP ( 'NONE', ( #18781, #8487, #12413, #10334 ) ) ;
#2045=AXIS2_PLACEMENT_3D ( 'NONE', #5376, #13213, #11549 ) ;
#2053=ORIENTED_EDGE ( 'NONE', *, *, #13953, .F. ) ;
#2055=ORIENTED_EDGE ( 'NONE', *, *, #2145, .T. ) ;
#2057=VECTOR ( 'NONE', #20111, 1000.000000000000000 ) ;
#2060=DIRECTION ( 'NONE',  ( -0.000000000000000000, -0.000000000000000000, -1.000000000000000000 ) ) ;
#2061=EDGE_CURVE ( 'NONE', #12082, #18231, #10892, .T. ) ;
#2064=DIRECTION ( 'NONE',  ( 1.000000000000000000, 0.000000000000000000, 0.000000000000000000 ) ) ;
#2066=EDGE_CURVE ( 'NONE', #16093, #15361, #20622, .T. ) ;
#2068=CARTESIAN_POINT ( 'NONE',  ( -13.81494360078803396, 11.64110105645932691, 10.00000000000000000 ) ) ;
#2070=AXIS2_PLACEMENT_3D ( 'NONE', #12017, #835, #5643 ) ;
#2077=DIRECTION ( 'NONE',  ( 0.000000000000000000, 0.000000000000000000, 1.000000000000000000 ) ) ;
#2078=ORIENTED_EDGE ( 'NONE', *, *, #18843, .T. ) ;
#2084=AXIS2_PLACEMENT_3D ( 'NONE', #16790, #18162, #16482 ) ;
#2086=EDGE_CURVE ( 'NONE', #19354, #13385, #1676, .T. ) ;
#2094=DIRECTION ( 'NONE',  ( 0.000000000000000000, 0.000000000000000000, -1.000000000000000000 ) ) ;
#2095=FACE_OUTER_BOUND ( 'NONE', #234, .T. ) ;
#2099=ORIENTED_EDGE ( 'NONE', *, *, #338, .F. ) ;
#2113=DIRECTION ( 'NONE',  ( 0.000000000000000000, 1.000000000000000000, -0.000000000000000000 ) ) ;
#2123=ORIENTED_EDGE ( 'NONE', *, *, #13146, .T. ) ;
#2131=ADVANCED_FACE ( 'NONE', ( #17256 ), #11193, .T. ) ;
#2132=EDGE_CURVE ( 'NONE', #15823, #3062, #2935, .T. ) ;
#2133=DIRECTION ( 'NONE',  ( -1.000000000000000000, 0.000000000000000000, 0.000000000000000000 ) ) ;
#2134=PLANE ( 'NONE',  #13664 ) ;
#2137=DIRECTION ( 'NONE',  ( 1.000000000000000000, 0.000000000000000000, -0.000000000000000000 ) ) ;
#2139=DIRECTION ( 'NONE',  ( 0.000000000000000000, -1.000000000000000000, 0.000000000000000000 ) ) ;
#2145=EDGE_CURVE ( 'NONE', #15521, #3725, #3146, .T. ) ;
#2152=LINE ( 'NONE', #11255, #11386 ) ;
#2153=ORIENTED_EDGE ( 'NONE', *, *, #2460, .F. ) ;
#2155=ORIENTED_EDGE ( 'NONE', *, *, #8173, .T. ) ;
#2170=VERTEX_POINT ( 'NONE', #17570 ) ;
#2172=DIRECTION ( 'NONE',  ( -0.000000000000000000, 0.000000000000000000, -1.000000000000000000 ) ) ;
#2173=PLANE ( 'NONE',  #15347 ) ;
#2174=ORIENTED_EDGE ( 'NONE', *, *, #4992, .T. ) ;
#2175=ORIENTED_EDGE ( 'NONE', *, *, #4062, .T. ) ;
#2179=ORIENTED_EDGE ( 'NONE', *, *, #14452, .F. ) ;
#2183=DIRECTION ( 'NONE',  ( 0.000000000000000000, 0.000000000000000000, 1.000000000000000000 ) ) ;
#2184=CARTESIAN_POINT ( 'NONE',  ( -0.000000000000000000, 11.64110105645932691, 0.000000000000000000 ) ) ;
#2191=CARTESIAN_POINT ( 'NONE',  ( -0.1250000000000001110, 0.000000000000000000, 1.000000000000000000 ) ) ;
#2193=EDGE_CURVE ( 'NONE', #7935, #12082, #20718, .T. ) ;
#2197=ORIENTED_EDGE ( 'NONE', *, *, #13364, .T. ) ;
#2204=EDGE_CURVE ( 'NONE', #3058, #16093, #14214, .T. ) ;
#2213=DIRECTION ( 'NONE',  ( 1.000000000000000000, -0.000000000000000000, 0.000000000000000000 ) ) ;
#2223=VECTOR ( 'NONE', #15836, 1000.000000000000000 ) ;
#2224=FACE_OUTER_BOUND ( 'NONE', #1017, .T. ) ;
#2230=FACE_OUTER_BOUND ( 'NONE', #17720, .T. ) ;
#2233=DIRECTION ( 'NONE',  ( -0.000000000000000000, 0.000000000000000000, -1.000000000000000000 ) ) ;
#2243=ORIENTED_EDGE ( 'NONE', *, *, #4992, .F. ) ;
#2247=ORIENTED_EDGE ( 'NONE', *, *, #4115, .T. ) ;
#2249=CARTESIAN_POINT ( 'NONE',  ( -10.43924542913431175, 0.000000000000000000, 0.000000000000000000 ) ) ;
#2252=EDGE_LOOP ( 'NONE', ( #11663, #6423, #14103, #14980 ) ) ;
#2260=CARTESIAN_POINT ( 'NONE',  ( -17.94064177244175795, 0.000000000000000000, 1.000000000000000000 ) ) ;
#2265=ORIENTED_EDGE ( 'NONE', *, *, #16645, .F. ) ;
#2282=LINE ( 'NONE', #8672, #3826 ) ;
#2284=DIRECTION ( 'NONE',  ( 0.000000000000000000, 1.000000000000000000, -0.000000000000000000 ) ) ;
#2290=DIRECTION ( 'NONE',  ( 1.000000000000000000, 0.000000000000000000, 0.000000000000000000 ) ) ;
#2295=VECTOR ( 'NONE', #5825, 1000.000000000000000 ) ;
#2299=CARTESIAN_POINT ( 'NONE',  ( -14.56494360078803396, 0.000000000000000000, 1.000000000000000000 ) ) ;
#2300=ORIENTED_EDGE ( 'NONE', *, *, #12681, .T. ) ;
#2302=DIRECTION ( 'NONE',  ( -0.000000000000000000, -0.000000000000000000, -1.000000000000000000 ) ) ;
#2305=VECTOR ( 'NONE', #12289, 1000.000000000000000 ) ;
#2307=AXIS2_PLACEMENT_3D ( 'NONE', #13236, #11476, #5291 ) ;
#2309=ADVANCED_FACE ( 'NONE', ( #9829 ), #11700, .T. ) ;
#2311=LINE ( 'NONE', #16438, #17401 ) ;
#2316=EDGE_CURVE ( 'NONE', #7608, #1742, #18098, .T. ) ;
#2324=DIRECTION ( 'NONE',  ( 0.000000000000000000, 0.000000000000000000, -1.000000000000000000 ) ) ;
#2325=ORIENTED_EDGE ( 'NONE', *, *, #19639, .F. ) ;
#2331=CARTESIAN_POINT ( 'NONE',  ( -20.75349085826862350, 11.64110105645932691, 10.00000000000000000 ) ) ;
#2338=CARTESIAN_POINT ( 'NONE',  ( -26.19203811574920593, 11.64110105645932691, 0.000000000000000000 ) ) ;
#2342=ORIENTED_EDGE ( 'NONE', *, *, #2552, .T. ) ;
#2345=AXIS2_PLACEMENT_3D ( 'NONE', #13280, #10258, #18214 ) ;
#2348=ORIENTED_EDGE ( 'NONE', *, *, #6891, .F. ) ;
#2351=ORIENTED_EDGE ( 'NONE', *, *, #5064, .F. ) ;
#2357=EDGE_LOOP ( 'NONE', ( #4842, #13020, #8609, #10338 ) ) ;
#2361=VECTOR ( 'NONE', #11432, 1000.000000000000000 ) ;
#2363=VECTOR ( 'NONE', #7257, 1000.000000000000000 ) ;
#2368=AXIS2_PLACEMENT_3D ( 'NONE', #5168, #11450, #13524 ) ;
#2372=CARTESIAN_POINT ( 'NONE',  ( 0.000000000000000000, 11.64110105645932691, 10.00000000000000000 ) ) ;
#2375=ORIENTED_EDGE ( 'NONE', *, *, #13312, .F. ) ;
#2380=CARTESIAN_POINT ( 'NONE',  ( -20.75349085826862350, 10.00000000000000000, 0.000000000000000000 ) ) ;
#2384=ORIENTED_EDGE ( 'NONE', *, *, #12976, .F. ) ;
#2386=CARTESIAN_POINT ( 'NONE',  ( 6.813547257480585095, 16.00000000000000000, 1.000000000000000000 ) ) ;
#2391=DIRECTION ( 'NONE',  ( 0.000000000000000000, 1.000000000000000000, -0.000000000000000000 ) ) ;
#2392=VECTOR ( 'NONE', #17653, 1000.000000000000000 ) ;
#2404=CARTESIAN_POINT ( 'NONE',  ( -1.437849085826860884, 11.64110105645932691, 10.00000000000000000 ) ) ;
#2405=EDGE_LOOP ( 'NONE', ( #11894, #6714, #11003, #19452 ) ) ;
#2409=VERTEX_POINT ( 'NONE', #14939 ) ;
#2417=PLANE ( 'NONE',  #1043 ) ;
#2422=VECTOR ( 'NONE', #3088, 1000.000000000000000 ) ;
#2427=ORIENTED_EDGE ( 'NONE', *, *, #19253, .T. ) ;
#2431=ORIENTED_EDGE ( 'NONE', *, *, #4015, .T. ) ;
#2435=AXIS2_PLACEMENT_3D ( 'NONE', #12950, #14735, #19767 ) ;
#2436=CARTESIAN_POINT ( 'NONE',  ( 6.063547257480584207, 0.000000000000000000, 0.000000000000000000 ) ) ;
#2440=DIRECTION ( 'NONE',  ( 1.000000000000000000, 0.000000000000000000, -0.000000000000000000 ) ) ;
#2442=CARTESIAN_POINT ( 'NONE',  ( -14.56494360078803396, 16.00000000000000000, 1.000000000000000000 ) ) ;
#2445=VERTEX_POINT ( 'NONE', #10238 ) ;
#2450=ORIENTED_EDGE ( 'NONE', *, *, #15273, .T. ) ;
#2452=LINE ( 'NONE', #789, #14727 ) ;
#2460=EDGE_CURVE ( 'NONE', #7326, #20051, #16369, .T. ) ;
#2463=DIRECTION ( 'NONE',  ( 1.000000000000000000, -0.000000000000000000, 0.000000000000000000 ) ) ;
#2466=CARTESIAN_POINT ( 'NONE',  ( 0.000000000000000000, 11.64110105645932691, 0.000000000000000000 ) ) ;
#2471=DIRECTION ( 'NONE',  ( 1.000000000000000000, -0.000000000000000000, 0.000000000000000000 ) ) ;
#2480=DIRECTION ( 'NONE',  ( 1.000000000000000000, 0.000000000000000000, 0.000000000000000000 ) ) ;
#2481=VERTEX_POINT ( 'NONE', #12318 ) ;
#2482=VERTEX_POINT ( 'NONE', #7113 ) ;
#2493=EDGE_LOOP ( 'NONE', ( #630, #1999, #10925, #15522 ) ) ;
#2502=ORIENTED_EDGE ( 'NONE', *, *, #338, .T. ) ;
#2504=VECTOR ( 'NONE', #11042, 1000.000000000000000 ) ;
#2505=CARTESIAN_POINT ( 'NONE',  ( -0.000000000000000000, 11.64110105645932691, 0.000000000000000000 ) ) ;
#2509=PLANE ( 'NONE',  #2345 ) ;
#2516=DIRECTION ( 'NONE',  ( -1.156482317317871331E-15, 1.000000000000000000, -0.000000000000000000 ) ) ;
#2527=CYLINDRICAL_SURFACE ( 'NONE', #12346, 10.00000000000000000 ) ;
#2532=CIRCLE ( 'NONE', #10562, 10.00000000000000000 ) ;
#2536=EDGE_CURVE ( 'NONE', #15304, #15313, #10456, .T. ) ;
#2537=DIRECTION ( 'NONE',  ( 0.000000000000000000, 1.000000000000000000, -0.000000000000000000 ) ) ;
#2539=CARTESIAN_POINT ( 'NONE',  ( 13.00209451496117374, 16.00000000000000000, 1.000000000000000000 ) ) ;
#2548=DIRECTION ( 'NONE',  ( -1.000000000000000000, -1.156482317317871133E-15, 0.000000000000000000 ) ) ;
#2552=EDGE_CURVE ( 'NONE', #12182, #7127, #19879, .T. ) ;
#2558=ORIENTED_EDGE ( 'NONE', *, *, #15684, .F. ) ;
#2560=CIRCLE ( 'NONE', #4240, 10.00000000000000000 ) ;
#2562=DIRECTION ( 'NONE',  ( 0.000000000000000000, -1.000000000000000000, 0.000000000000000000 ) ) ;
#2570=DIRECTION ( 'NONE',  ( -1.000000000000000000, -1.156482317317871725E-16, -0.000000000000000000 ) ) ;
#2573=LINE ( 'NONE', #12099, #8892 ) ;
#2580=VERTEX_POINT ( 'NONE', #19976 ) ;
#2581=AXIS2_PLACEMENT_3D ( 'NONE', #1064, #13594, #13906 ) ;
#2584=LINE ( 'NONE', #9660, #5003 ) ;
#2588=ORIENTED_EDGE ( 'NONE', *, *, #1207, .T. ) ;
#2592=CARTESIAN_POINT ( 'NONE',  ( 8.876396343307449754, 10.00000000000000000, 1.000000000000000000 ) ) ;
#2594=VECTOR ( 'NONE', #4166, 1000.000000000000000 ) ;
#2606=ORIENTED_EDGE ( 'NONE', *, *, #11830, .T. ) ;
#2609=CARTESIAN_POINT ( 'NONE',  ( -5.563547257480587760, 0.000000000000000000, 0.000000000000000000 ) ) ;
#2616=CARTESIAN_POINT ( 'NONE',  ( 22.56633994409548194, 10.00000000000000000, 0.000000000000000000 ) ) ;
#2619=EDGE_CURVE ( 'NONE', #13746, #4108, #3958, .T. ) ;
#2620=EDGE_CURVE ( 'NONE', #15262, #2170, #13674, .T. ) ;
#2621=DIRECTION ( 'NONE',  ( 0.000000000000000000, -1.000000000000000000, 0.000000000000000000 ) ) ;
#2625=LINE ( 'NONE', #4410, #19437 ) ;
#2631=AXIS2_PLACEMENT_3D ( 'NONE', #12717, #13973, #6041 ) ;
#2634=ORIENTED_EDGE ( 'NONE', *, *, #2145, .F. ) ;
#2637=ORIENTED_EDGE ( 'NONE', *, *, #1172, .T. ) ;
#2638=EDGE_CURVE ( 'NONE', #2482, #2481, #16717, .T. ) ;
#2639=VERTEX_POINT ( 'NONE', #16922 ) ;
#2640=LINE ( 'NONE', #20127, #14451 ) ;
#2649=CARTESIAN_POINT ( 'NONE',  ( -9.000000000000000000, -9.999999999999992895, 2.000000000000000000 ) ) ;
#2650=CARTESIAN_POINT ( 'NONE',  ( -18.69064177244175795, 0.000000000000000000, 0.000000000000000000 ) ) ;
#2652=CIRCLE ( 'NONE', #18354, 10.00000000000000000 ) ;
#2654=VERTEX_POINT ( 'NONE', #5850 ) ;
#2663=VERTEX_POINT ( 'NONE', #1144 ) ;
#2665=EDGE_CURVE ( 'NONE', #3979, #932, #13886, .T. ) ;
#2668=ORIENTED_EDGE ( 'NONE', *, *, #17168, .T. ) ;
#2672=ORIENTED_EDGE ( 'NONE', *, *, #20182, .T. ) ;
#2674=CARTESIAN_POINT ( 'NONE',  ( -30.00000000000000000, 0.000000000000000000, 0.000000000000000000 ) ) ;
#2676=LINE ( 'NONE', #7395, #17000 ) ;
#2678=FACE_OUTER_BOUND ( 'NONE', #15058, .T. ) ;
#2679=AXIS2_PLACEMENT_3D ( 'NONE', #18016, #10170, #16540 ) ;
#2682=DIRECTION ( 'NONE',  ( 0.000000000000000000, 1.000000000000000000, 0.000000000000000000 ) ) ;
#2688=EDGE_LOOP ( 'NONE', ( #1022, #19401, #17815, #17406 ) ) ;
#2692=EDGE_LOOP ( 'NONE', ( #16128, #8297 ) ) ;
#2693=DIRECTION ( 'NONE',  ( -0.000000000000000000, -0.000000000000000000, -1.000000000000000000 ) ) ;
#2700=VERTEX_POINT ( 'NONE', #9880 ) ;
#2705=CARTESIAN_POINT ( 'NONE',  ( 6.813547257480585095, 0.000000000000000000, 0.000000000000000000 ) ) ;
#2708=CARTESIAN_POINT ( 'NONE',  ( -13.81494360078803396, 0.000000000000000000, 1.000000000000000000 ) ) ;
#2716=CARTESIAN_POINT ( 'NONE',  ( -5.563547257480587760, 16.00000000000000000, 1.000000000000000000 ) ) ;
#2720=ORIENTED_EDGE ( 'NONE', *, *, #2961, .F. ) ;
#2723=LINE ( 'NONE', #2505, #9466 ) ;
#2724=VERTEX_POINT ( 'NONE', #9474 ) ;
#2729=AXIS2_PLACEMENT_3D ( 'NONE', #4531, #4734, #1398 ) ;
#2736=DIRECTION ( 'NONE',  ( -1.000000000000000000, 0.000000000000000000, 0.000000000000000000 ) ) ;
#2738=CARTESIAN_POINT ( 'NONE',  ( -0.000000000000000000, 11.64110105645932691, 0.000000000000000000 ) ) ;
#2747=DIRECTION ( 'NONE',  ( 1.000000000000000000, 0.000000000000000000, 0.000000000000000000 ) ) ;
#2753=AXIS2_PLACEMENT_3D ( 'NONE', #11611, #14951, #327 ) ;
#2755=LINE ( 'NONE', #4114, #17659 ) ;
#2759=DIRECTION ( 'NONE',  ( -0.000000000000000000, -0.000000000000000000, -1.000000000000000000 ) ) ;
#2760=CARTESIAN_POINT ( 'NONE',  ( 0.000000000000000000, 10.00000000000000000, 1.000000000000000000 ) ) ;
#2762=FACE_OUTER_BOUND ( 'NONE', #2044, .T. ) ;
#2773=ORIENTED_EDGE ( 'NONE', *, *, #18228, .F. ) ;
#2774=ORIENTED_EDGE ( 'NONE', *, *, #1366, .F. ) ;
#2776=DIRECTION ( 'NONE',  ( 0.000000000000000000, 1.000000000000000000, -0.000000000000000000 ) ) ;
#2782=EDGE_LOOP ( 'NONE', ( #13086, #10053, #16818, #6268 ) ) ;
#2786=CARTESIAN_POINT ( 'NONE',  ( -16.62779268661489951, 0.000000000000000000, 1.000000000000000000 ) ) ;
#2788=CARTESIAN_POINT ( 'NONE',  ( 0.000000000000000000, 10.00000000000000000, 1.000000000000000000 ) ) ;
#2793=DIRECTION ( 'NONE',  ( -0.000000000000000000, 0.000000000000000000, -1.000000000000000000 ) ) ;
#2801=CARTESIAN_POINT ( 'NONE',  ( 0.000000000000000000, 16.00000000000000000, 1.000000000000000000 ) ) ;
#2803=CARTESIAN_POINT ( 'NONE',  ( 6.813547257480585095, 0.000000000000000000, 1.000000000000000000 ) ) ;
#2807=DIRECTION ( 'NONE',  ( 0.000000000000000000, -1.000000000000000000, 0.000000000000000000 ) ) ;
#2808=LINE ( 'NONE', #1238, #13965 ) ;
#2817=EDGE_CURVE ( 'NONE', #14753, #13, #4762, .T. ) ;
#2820=DIRECTION ( 'NONE',  ( -0.000000000000000000, -0.000000000000000000, -1.000000000000000000 ) ) ;
#2830=VERTEX_POINT ( 'NONE', #17516 ) ;
#2837=CARTESIAN_POINT ( 'NONE',  ( 14.99999999999999645, 3.000000000000003553, 1.000000000000000000 ) ) ;
#2841=DIRECTION ( 'NONE',  ( 0.000000000000000000, 0.000000000000000000, -1.000000000000000000 ) ) ;
#2849=EDGE_CURVE ( 'NONE', #8796, #11652, #12810, .T. ) ;
#2851=ORIENTED_EDGE ( 'NONE', *, *, #6596, .T. ) ;
#2860=FACE_OUTER_BOUND ( 'NONE', #2405, .T. ) ;
#2862=DIRECTION ( 'NONE',  ( -0.000000000000000000, 0.000000000000000000, -1.000000000000000000 ) ) ;
#2867=FACE_OUTER_BOUND ( 'NONE', #15855, .T. ) ;
#2874=ORIENTED_EDGE ( 'NONE', *, *, #3496, .F. ) ;
#2876=ORIENTED_EDGE ( 'NONE', *, *, #2665, .T. ) ;
#2879=LINE ( 'NONE', #13951, #13466 ) ;
#2880=ORIENTED_EDGE ( 'NONE', *, *, #13846, .F. ) ;
#2885=LINE ( 'NONE', #2788, #5518 ) ;
#2888=DIRECTION ( 'NONE',  ( 0.1736481776669309696, 0.9848077530122080203, 0.000000000000000000 ) ) ;
#2897=EDGE_LOOP ( 'NONE', ( #11589, #6623, #19194, #16123 ) ) ;
#2899=CYLINDRICAL_SURFACE ( 'NONE', #2631, 10.00000000000000000 ) ;
#2900=VERTEX_POINT ( 'NONE', #18038 ) ;
#2901=LINE ( 'NONE', #2803, #17321 ) ;
#2902=ORIENTED_EDGE ( 'NONE', *, *, #20416, .F. ) ;
#2912=DIRECTION ( 'NONE',  ( 0.000000000000000000, -1.000000000000000000, 0.000000000000000000 ) ) ;
#2917=VERTEX_POINT ( 'NONE', #2338 ) ;
#2921=ORIENTED_EDGE ( 'NONE', *, *, #1772, .F. ) ;
#2924=VERTEX_POINT ( 'NONE', #11855 ) ;
#2928=EDGE_CURVE ( 'NONE', #7935, #20454, #567, .T. ) ;
#2930=VERTEX_POINT ( 'NONE', #8732 ) ;
#2935=LINE ( 'NONE', #15691, #2009 ) ;
#2943=CIRCLE ( 'NONE', #10308, 10.00000000000000000 ) ;
#2948=UNCERTAINTY_MEASURE_WITH_UNIT (LENGTH_MEASURE( 1.000000000000000082E-05 ), #5234, 'distance_accuracy_value', 'NONE');
#2950=LINE ( 'NONE', #14229, #6777 ) ;
#2957=EDGE_CURVE ( 'NONE', #3619, #886, #14033, .T. ) ;
#2958=CARTESIAN_POINT ( 'NONE',  ( 30.80549002841696904, 5.431839045955454637, 1.000000000000000000 ) ) ;
#2961=EDGE_CURVE ( 'NONE', #10855, #3441, #20405, .T. ) ;
#2964=AXIS2_PLACEMENT_3D ( 'NONE', #6145, #12415, #12515 ) ;
#2969=CARTESIAN_POINT ( 'NONE',  ( 0.000000000000000000, 0.000000000000000000, 1.000000000000000000 ) ) ;
#2972=EDGE_LOOP ( 'NONE', ( #18261, #1789, #16206, #1304 ) ) ;
#2979=CARTESIAN_POINT ( 'NONE',  ( 0.000000000000000000, 10.00000000000000000, 1.000000000000000000 ) ) ;
#2981=EDGE_LOOP ( 'NONE', ( #14500, #6094, #12941, #13436 ) ) ;
#2983=EDGE_CURVE ( 'NONE', #15823, #9991, #11518, .T. ) ;
#2994=CARTESIAN_POINT ( 'NONE',  ( -27.00000000000000000, 0.000000000000000000, 1.000000000000000000 ) ) ;
#3004=FACE_OUTER_BOUND ( 'NONE', #7410, .T. ) ;
#3005=ORIENTED_EDGE ( 'NONE', *, *, #3962, .T. ) ;
#3009=VECTOR ( 'NONE', #1517, 1000.000000000000000 ) ;
#3013=ORIENTED_EDGE ( 'NONE', *, *, #13364, .F. ) ;
#3023=DIRECTION ( 'NONE',  ( 0.000000000000000000, -0.000000000000000000, 1.000000000000000000 ) ) ;
#3025=ORIENTED_EDGE ( 'NONE', *, *, #14321, .F. ) ;
#3030=AXIS2_PLACEMENT_3D ( 'NONE', #7133, #4089, #15267 ) ;
#3032=CARTESIAN_POINT ( 'NONE',  ( -14.56494360078803396, 10.00000000000000000, 1.000000000000000000 ) ) ;
#3047=VECTOR ( 'NONE', #16037, 1000.000000000000114 ) ;
#3048=CIRCLE ( 'NONE', #20424, 10.00000000000000000 ) ;
#3049=DIRECTION ( 'NONE',  ( -0.000000000000000000, -0.000000000000000000, -1.000000000000000000 ) ) ;
#3058=VERTEX_POINT ( 'NONE', #6514 ) ;
#3062=VERTEX_POINT ( 'NONE', #333 ) ;
#3071=CARTESIAN_POINT ( 'NONE',  ( 15.06494360078803041, 0.000000000000000000, 0.000000000000000000 ) ) ;
#3076=ORIENTED_EDGE ( 'NONE', *, *, #16276, .F. ) ;
#3079=EDGE_CURVE ( 'NONE', #7127, #7382, #17721, .T. ) ;
#3082=ORIENTED_EDGE ( 'NONE', *, *, #8366, .T. ) ;
#3088=DIRECTION ( 'NONE',  ( 1.000000000000000000, 0.000000000000000000, 0.000000000000000000 ) ) ;
#3091=ORIENTED_EDGE ( 'NONE', *, *, #8983, .T. ) ;
#3094=DIRECTION ( 'NONE',  ( 0.000000000000000000, 1.000000000000000000, 0.000000000000000000 ) ) ;
#3097=DIRECTION ( 'NONE',  ( 1.000000000000000000, -0.000000000000000000, 0.000000000000000000 ) ) ;
#3104=CIRCLE ( 'NONE', #14784, 10.00000000000000000 ) ;
#3110=EDGE_LOOP ( 'NONE', ( #5314, #11766, #10025, #5704 ) ) ;
#3114=EDGE_CURVE ( 'NONE', #12054, #5420, #19069, .T. ) ;
#3116=ORIENTED_EDGE ( 'NONE', *, *, #18821, .T. ) ;
#3127=EDGE_CURVE ( 'NONE', #12822, #9362, #11212, .T. ) ;
#3131=ORIENTED_EDGE ( 'NONE', *, *, #7199, .F. ) ;
#3138=CARTESIAN_POINT ( 'NONE',  ( -1.734723475976795735E-14, 10.00000000000004619, 0.000000000000000000 ) ) ;
#3146=LINE ( 'NONE', #12647, #5008 ) ;
#3151=ADVANCED_FACE ( 'NONE', ( #9748 ), #223, .T. ) ;
#3152=FACE_OUTER_BOUND ( 'NONE', #4829, .T. ) ;
#3160=ORIENTED_EDGE ( 'NONE', *, *, #1682, .F. ) ;
#3168=CARTESIAN_POINT ( 'NONE',  ( -2.187849085826861550, 16.00000000000000000, 1.000000000000000000 ) ) ;
#3172=CARTESIAN_POINT ( 'NONE',  ( -30.80549002841696193, 5.431839045955507927, 0.000000000000000000 ) ) ;
#3177=CARTESIAN_POINT ( 'NONE',  ( 10.18924542913430820, 10.00000000000000000, 0.000000000000000000 ) ) ;
#3192=VECTOR ( 'NONE', #7285, 1000.000000000000000 ) ;
#3193=CARTESIAN_POINT ( 'NONE',  ( 14.31494360078803041, 0.000000000000000000, 1.000000000000000000 ) ) ;
#3208=DIRECTION ( 'NONE',  ( -1.000000000000000000, 0.000000000000000000, 0.000000000000000000 ) ) ;
#3211=DIRECTION ( 'NONE',  ( 0.000000000000000000, 0.000000000000000000, -1.000000000000000000 ) ) ;
#3218=DIRECTION ( 'NONE',  ( -0.000000000000000000, -0.000000000000000000, -1.000000000000000000 ) ) ;
#3220=LINE ( 'NONE', #9702, #11950 ) ;
#3225=ORIENTED_EDGE ( 'NONE', *, *, #5453, .F. ) ;
#3229=ORIENTED_EDGE ( 'NONE', *, *, #409, .T. ) ;
#3239=ADVANCED_FACE ( 'NONE', ( #8490 ), #5452, .T. ) ;
#3242=DIRECTION ( 'NONE',  ( 0.000000000000000000, 0.000000000000000000, 1.000000000000000000 ) ) ;
#3249=VECTOR ( 'NONE', #10570, 1000.000000000000000 ) ;
#3250=EDGE_CURVE ( 'NONE', #13, #5953, #534, .T. ) ;
#3253=VERTEX_POINT ( 'NONE', #13592 ) ;
#3256=DIRECTION ( 'NONE',  ( 1.000000000000000000, -0.000000000000000000, 0.000000000000000000 ) ) ;
#3258=ORIENTED_EDGE ( 'NONE', *, *, #5509, .T. ) ;
#3260=DIRECTION ( 'NONE',  ( 0.000000000000000000, 0.000000000000000000, -1.000000000000000000 ) ) ;
#3266=DIRECTION ( 'NONE',  ( -0.000000000000000000, -0.000000000000000000, -1.000000000000000000 ) ) ;
#3274=CARTESIAN_POINT ( 'NONE',  ( 0.000000000000000000, 16.00000000000000000, 1.000000000000000000 ) ) ;
#3281=EDGE_LOOP ( 'NONE', ( #3636, #7383, #3386, #18163 ) ) ;
#3283=CARTESIAN_POINT ( 'NONE',  ( -15.00000000000000000, 0.000000000000000000, 2.000000000000000000 ) ) ;
#3284=LINE ( 'NONE', #14255, #2223 ) ;
#3287=CARTESIAN_POINT ( 'NONE',  ( 0.000000000000000000, 10.00000000000000000, 1.000000000000000000 ) ) ;
#3292=LINE ( 'NONE', #15943, #17664 ) ;
#3300=ADVANCED_FACE ( 'NONE', ( #18424 ), #2509, .T. ) ;
#3303=ORIENTED_EDGE ( 'NONE', *, *, #12397, .F. ) ;
#3306=ORIENTED_EDGE ( 'NONE', *, *, #19763, .F. ) ;
#3308=ORIENTED_EDGE ( 'NONE', *, *, #6444, .T. ) ;
#3310=ORIENTED_EDGE ( 'NONE', *, *, #7828, .T. ) ;
#3331=CARTESIAN_POINT ( 'NONE',  ( -22.81633994409548549, 10.00000000000000000, 1.000000000000000000 ) ) ;
#3334=LINE ( 'NONE', #6379, #252 ) ;
#3341=ORIENTED_EDGE ( 'NONE', *, *, #15117, .T. ) ;
#3348=CARTESIAN_POINT ( 'NONE',  ( -0.000000000000000000, 11.64110105645932691, 0.000000000000000000 ) ) ;
#3352=VECTOR ( 'NONE', #8217, 1000.000000000000000 ) ;
#3355=EDGE_CURVE ( 'NONE', #17557, #5957, #7333, .T. ) ;
#3361=FACE_OUTER_BOUND ( 'NONE', #8272, .T. ) ;
#3362=ORIENTED_EDGE ( 'NONE', *, *, #6706, .T. ) ;
#3368=VECTOR ( 'NONE', #18881, 1000.000000000000000 ) ;
#3369=VECTOR ( 'NONE', #5055, 1000.000000000000000 ) ;
#3373=DIRECTION ( 'NONE',  ( -1.000000000000000000, 0.000000000000000000, 0.000000000000000000 ) ) ;
#3381=DIRECTION ( 'NONE',  ( 1.000000000000000000, 0.000000000000000000, 0.000000000000000000 ) ) ;
#3386=ORIENTED_EDGE ( 'NONE', *, *, #7138, .F. ) ;
#3392=VERTEX_POINT ( 'NONE', #8693 ) ;
#3394=CARTESIAN_POINT ( 'NONE',  ( 6.063547257480584207, 10.00000000000000000, 0.000000000000000000 ) ) ;
#3396=CIRCLE ( 'NONE', #73, 10.00000000000000000 ) ;
#3400=CARTESIAN_POINT ( 'NONE',  ( -4.250698171653726654, 11.64110105645932691, 0.000000000000000000 ) ) ;
#3401=CARTESIAN_POINT ( 'NONE',  ( -10.49999999999999822, -9.999999999999992895, 2.000000000000000000 ) ) ;
#3402=CARTESIAN_POINT ( 'NONE',  ( -5.563547257480587760, 10.00000000000000000, 1.000000000000000000 ) ) ;
#3410=EDGE_CURVE ( 'NONE', #17844, #2654, #680, .T. ) ;
#3429=CARTESIAN_POINT ( 'NONE',  ( 27.44203811574919882, 11.64110105645932691, 0.000000000000000000 ) ) ;
#3433=ORIENTED_EDGE ( 'NONE', *, *, #14900, .T. ) ;
#3438=CYLINDRICAL_SURFACE ( 'NONE', #8619, 10.00000000000000000 ) ;
#3440=ORIENTED_EDGE ( 'NONE', *, *, #18783, .F. ) ;
#3441=VERTEX_POINT ( 'NONE', #17211 ) ;
#3446=EDGE_CURVE ( 'NONE', #13746, #19940, #20264, .T. ) ;
#3457=CARTESIAN_POINT ( 'NONE',  ( -0.000000000000000000, 10.00000000000000000, 0.000000000000000000 ) ) ;
#3460=ORIENTED_EDGE ( 'NONE', *, *, #13953, .T. ) ;
#3463=PLANE ( 'NONE',  #9769 ) ;
#3466=AXIS2_PLACEMENT_3D ( 'NONE', #6909, #10154, #16525 ) ;
#3472=EDGE_CURVE ( 'NONE', #17017, #9770, #10530, .T. ) ;
#3474=AXIS2_PLACEMENT_3D ( 'NONE', #2760, #978, #9138 ) ;
#3479=CARTESIAN_POINT ( 'NONE',  ( 0.000000000000000000, 11.64110105645932691, 10.00000000000000000 ) ) ;
#3480=ADVANCED_FACE ( 'NONE', ( #10943 ), #4357, .T. ) ;
#3481=ORIENTED_EDGE ( 'NONE', *, *, #4137, .T. ) ;
#3487=ORIENTED_EDGE ( 'NONE', *, *, #1116, .T. ) ;
#3492=ORIENTED_EDGE ( 'NONE', *, *, #7758, .T. ) ;
#3493=DIRECTION ( 'NONE',  ( 0.000000000000000000, 1.000000000000000000, -0.000000000000000000 ) ) ;
#3496=EDGE_CURVE ( 'NONE', #16502, #9634, #23, .T. ) ;
#3497=LINE ( 'NONE', #9875, #11009 ) ;
#3499=LINE ( 'NONE', #1927, #12059 ) ;
#3513=ORIENTED_EDGE ( 'NONE', *, *, #11312, .T. ) ;
#3516=ORIENTED_EDGE ( 'NONE', *, *, #8231, .T. ) ;
#3518=UNCERTAINTY_MEASURE_WITH_UNIT (LENGTH_MEASURE( 1.000000000000000082E-05 ), #13277, 'distance_accuracy_value', 'NONE');
#3520=DIRECTION ( 'NONE',  ( -0.000000000000000000, -0.000000000000000000, -1.000000000000000000 ) ) ;
#3523=CARTESIAN_POINT ( 'NONE',  ( 0.6250000000000005551, 0.000000000000000000, 0.000000000000000000 ) ) ;
#3525=EDGE_CURVE ( 'NONE', #2170, #15304, #1427, .T. ) ;
#3527=CARTESIAN_POINT ( 'NONE',  ( -22.06633994409548194, 10.00000000000000000, 1.000000000000000000 ) ) ;
#3528=CARTESIAN_POINT ( 'NONE',  ( 0.000000000000000000, 16.00000000000000000, 1.000000000000000000 ) ) ;
#3529=EDGE_CURVE ( 'NONE', #1441, #3058, #6135, .T. ) ;
#3542=AXIS2_PLACEMENT_3D ( 'NONE', #2372, #2471, #7290 ) ;
#3543=ORIENTED_EDGE ( 'NONE', *, *, #10836, .T. ) ;
#3545=ORIENTED_EDGE ( 'NONE', *, *, #15013, .F. ) ;
#3564=SURFACE_STYLE_FILL_AREA ( #17897 ) ;
#3567=VECTOR ( 'NONE', #1725, 1000.000000000000000 ) ;
#3570=DIRECTION ( 'NONE',  ( -0.000000000000000000, -0.000000000000000000, -1.000000000000000000 ) ) ;
#3585=AXIS2_PLACEMENT_3D ( 'NONE', #412, #16710, #7206 ) ;
#3586=DIRECTION ( 'NONE',  ( -1.000000000000000000, 0.000000000000000000, 0.000000000000000000 ) ) ;
#3587=ORIENTED_EDGE ( 'NONE', *, *, #4669, .T. ) ;
#3588=ADVANCED_FACE ( 'NONE', ( #7808 ), #14170, .T. ) ;
#3590=LINE ( 'NONE', #7049, #4430 ) ;
#3591=LINE ( 'NONE', #2436, #1235 ) ;
#3597=DIRECTION ( 'NONE',  ( 1.000000000000000000, 0.000000000000000000, 0.000000000000000000 ) ) ;
#3604=EDGE_LOOP ( 'NONE', ( #7927, #20325, #18564, #7685 ) ) ;
#3614=EDGE_CURVE ( 'NONE', #6794, #5732, #20369, .T. ) ;
#3615=VECTOR ( 'NONE', #2888, 999.9999999999998863 ) ;
#3619=VERTEX_POINT ( 'NONE', #19420 ) ;
#3620=LINE ( 'NONE', #19439, #13333 ) ;
#3621=CARTESIAN_POINT ( 'NONE',  ( 6.813547257480585095, 10.00000000000000000, 1.000000000000000000 ) ) ;
#3622=FACE_OUTER_BOUND ( 'NONE', #19252, .T. ) ;
#3628=DIRECTION ( 'NONE',  ( 0.000000000000000000, 0.000000000000000000, 1.000000000000000000 ) ) ;
#3633=VERTEX_POINT ( 'NONE', #4967 ) ;
#3636=ORIENTED_EDGE ( 'NONE', *, *, #18506, .T. ) ;
#3637=CARTESIAN_POINT ( 'NONE',  ( 3.469446951953523943E-14, 10.00000000000009592, 1.000000000000000000 ) ) ;
#3642=VECTOR ( 'NONE', #4756, 1000.000000000000000 ) ;
#3645=VECTOR ( 'NONE', #12844, 1000.000000000000000 ) ;
#3646=LINE ( 'NONE', #11592, #10131 ) ;
#3648=LINE ( 'NONE', #14737, #13937 ) ;
#3650=DIRECTION ( 'NONE',  ( 1.000000000000000000, 0.000000000000000000, 0.000000000000000000 ) ) ;
#3658=AXIS2_PLACEMENT_3D ( 'NONE', #5342, #17799, #16015 ) ;
#3666=VERTEX_POINT ( 'NONE', #15944 ) ;
#3670=EDGE_LOOP ( 'NONE', ( #7744, #19537, #16011, #18474 ) ) ;
#3676=CARTESIAN_POINT ( 'NONE',  ( 0.000000000000000000, 16.00000000000000000, 1.000000000000000000 ) ) ;
#3678=AXIS2_PLACEMENT_3D ( 'NONE', #1230, #10749, #20686 ) ;
#3680=VECTOR ( 'NONE', #1930, 1000.000000000000000 ) ;
#3681=CARTESIAN_POINT ( 'NONE',  ( 8.876396343307449754, 11.64110105645932691, 10.00000000000000000 ) ) ;
#3684=DIRECTION ( 'NONE',  ( -0.000000000000000000, -0.000000000000000000, -1.000000000000000000 ) ) ;
#3691=ORIENTED_EDGE ( 'NONE', *, *, #8097, .F. ) ;
#3695=CARTESIAN_POINT ( 'NONE',  ( -3.500698171653725765, 0.000000000000000000, 1.000000000000000000 ) ) ;
#3700=DIRECTION ( 'NONE',  ( 1.000000000000000000, -0.000000000000000000, 0.000000000000000000 ) ) ;
#3703=CARTESIAN_POINT ( 'NONE',  ( 22.56633994409548194, 0.000000000000000000, 1.000000000000000000 ) ) ;
#3706=AXIS2_PLACEMENT_3D ( 'NONE', #14944, #19474, #320 ) ;
#3708=VECTOR ( 'NONE', #7576, 1000.000000000000000 ) ;
#3713=VECTOR ( 'NONE', #15793, 1000.000000000000000 ) ;
#3722=ORIENTED_EDGE ( 'NONE', *, *, #6216, .F. ) ;
#3725=VERTEX_POINT ( 'NONE', #19111 ) ;
#3727=AXIS2_PLACEMENT_3D ( 'NONE', #19572, #6901, #13269 ) ;
#3730=DIRECTION ( 'NONE',  ( 0.000000000000000000, -1.000000000000000000, 0.000000000000000000 ) ) ;
#3736=CARTESIAN_POINT ( 'NONE',  ( 22.56633994409548194, 10.00000000000000000, 1.000000000000000000 ) ) ;
#3738=DIRECTION ( 'NONE',  ( 0.000000000000000000, 1.000000000000000000, -0.000000000000000000 ) ) ;
#3740=AXIS2_PLACEMENT_3D ( 'NONE', #17989, #11404, #10244 ) ;
#3742=VERTEX_POINT ( 'NONE', #14896 ) ;
#3743=EDGE_CURVE ( 'NONE', #7302, #9844, #574, .T. ) ;
#3748=DIRECTION ( 'NONE',  ( 0.000000000000000000, 0.000000000000000000, -1.000000000000000000 ) ) ;
#3754=VERTEX_POINT ( 'NONE', #986 ) ;
#3760=CARTESIAN_POINT ( 'NONE',  ( -18.69064177244175795, 0.000000000000000000, 1.000000000000000000 ) ) ;
#3767=CARTESIAN_POINT ( 'NONE',  ( -16.62779268661489951, 10.00000000000000000, 1.000000000000000000 ) ) ;
#3768=PLANE ( 'NONE',  #1073 ) ;
#3771=DIRECTION ( 'NONE',  ( -0.000000000000000000, -1.000000000000000000, -0.000000000000000000 ) ) ;
#3777=EDGE_LOOP ( 'NONE', ( #966, #3225, #1660, #17269 ) ) ;
#3778=EDGE_CURVE ( 'NONE', #18372, #5957, #10606, .T. ) ;
#3785=AXIS2_PLACEMENT_3D ( 'NONE', #4645, #18788, #11039 ) ;
#3788=DIRECTION ( 'NONE',  ( 1.000000000000000000, 0.000000000000000000, -0.000000000000000000 ) ) ;
#3802=EDGE_CURVE ( 'NONE', #2580, #14057, #10825, .T. ) ;
#3803=ORIENTED_EDGE ( 'NONE', *, *, #9135, .F. ) ;
#3806=CARTESIAN_POINT ( 'NONE',  ( 20.50349085826861995, 10.00000000000000000, 1.000000000000000000 ) ) ;
#3807=DIRECTION ( 'NONE',  ( 1.000000000000000000, -0.000000000000000000, 0.000000000000000000 ) ) ;
#3819=ORIENTED_EDGE ( 'NONE', *, *, #11460, .F. ) ;
#3821=DIRECTION ( 'NONE',  ( -1.000000000000000000, 0.000000000000000000, 0.000000000000000000 ) ) ;
#3824=ADVANCED_FACE ( 'NONE', ( #13939 ), #15515, .T. ) ;
#3826=VECTOR ( 'NONE', #19876, 1000.000000000000000 ) ;
#3827=ORIENTED_EDGE ( 'NONE', *, *, #7357, .F. ) ;
#3843=ORIENTED_EDGE ( 'NONE', *, *, #8470, .F. ) ;
#3847=ORIENTED_EDGE ( 'NONE', *, *, #5836, .T. ) ;
#3848=ORIENTED_EDGE ( 'NONE', *, *, #4115, .F. ) ;
#3849=EDGE_CURVE ( 'NONE', #17667, #3253, #6208, .T. ) ;
#3855=EDGE_CURVE ( 'NONE', #14060, #17851, #39, .T. ) ;
#3858=DIRECTION ( 'NONE',  ( -0.1736481776669309696, -0.9848077530122080203, 0.000000000000000000 ) ) ;
#3859=ADVANCED_FACE ( 'NONE', ( #2867 ), #18876, .T. ) ;
#3867=LINE ( 'NONE', #10148, #6079 ) ;
#3869=CARTESIAN_POINT ( 'NONE',  ( 16.37779268661489596, 10.00000000000000000, 1.000000000000000000 ) ) ;
#3875=VERTEX_POINT ( 'NONE', #15306 ) ;
#3883=DIRECTION ( 'NONE',  ( 1.000000000000000000, 0.000000000000000000, 0.000000000000000000 ) ) ;
#3904=DIRECTION ( 'NONE',  ( 0.000000000000000000, 0.000000000000000000, -1.000000000000000000 ) ) ;
#3906=LINE ( 'NONE', #13211, #19685 ) ;
#3908=FACE_OUTER_BOUND ( 'NONE', #19980, .T. ) ;
#3909=CARTESIAN_POINT ( 'NONE',  ( 10.93924542913430820, 11.64110105645932691, 0.000000000000000000 ) ) ;
#3926=DIRECTION ( 'NONE',  ( 1.000000000000000000, 0.000000000000000000, 0.000000000000000000 ) ) ;
#3948=ORIENTED_EDGE ( 'NONE', *, *, #2086, .T. ) ;
#3949=ORIENTED_EDGE ( 'NONE', *, *, #7074, .F. ) ;
#3951=ORIENTED_EDGE ( 'NONE', *, *, #20374, .F. ) ;
#3958=LINE ( 'NONE', #13785, #17366 ) ;
#3962=EDGE_CURVE ( 'NONE', #8358, #6555, #17735, .T. ) ;
#3967=AXIS2_PLACEMENT_3D ( 'NONE', #12061, #772, #873 ) ;
#3973=ORIENTED_EDGE ( 'NONE', *, *, #6288, .F. ) ;
#3975=ADVANCED_FACE ( 'NONE', ( #1812 ), #18978, .F. ) ;
#3977=PLANE ( 'NONE',  #14104 ) ;
#3979=VERTEX_POINT ( 'NONE', #11127 ) ;
#3984=CIRCLE ( 'NONE', #9331, 10.00000000000000000 ) ;
#3988=PLANE ( 'NONE',  #20089 ) ;
#4000=EDGE_CURVE ( 'NONE', #1851, #18752, #12683, .T. ) ;
#4003=CARTESIAN_POINT ( 'NONE',  ( -0.000000000000000000, 11.64110105645932691, 0.000000000000000000 ) ) ;
#4005=VECTOR ( 'NONE', #12253, 1000.000000000000000 ) ;
#4009=CARTESIAN_POINT ( 'NONE',  ( 2.687849085826861995, 11.64110105645932691, 0.000000000000000000 ) ) ;
#4015=EDGE_CURVE ( 'NONE', #2409, #8973, #19397, .T. ) ;
#4016=AXIS2_PLACEMENT_3D ( 'NONE', #11717, #19274, #8486 ) ;
#4039=DIRECTION ( 'NONE',  ( 0.000000000000000000, 0.000000000000000000, -1.000000000000000000 ) ) ;
#4040=AXIS2_PLACEMENT_3D ( 'NONE', #1502, #11325, #12788 ) ;
#4041=CIRCLE ( 'NONE', #17739, 10.00000000000000000 ) ;
#4044=CARTESIAN_POINT ( 'NONE',  ( -0.000000000000000000, 11.64110105645932691, 0.000000000000000000 ) ) ;
#4045=EDGE_CURVE ( 'NONE', #3619, #7837, #12577, .T. ) ;
#4053=VERTEX_POINT ( 'NONE', #6309 ) ;
#4056=ORIENTED_EDGE ( 'NONE', *, *, #20680, .T. ) ;
#4060=ORIENTED_EDGE ( 'NONE', *, *, #13780, .T. ) ;
#4062=EDGE_CURVE ( 'NONE', #20665, #10724, #19190, .T. ) ;
#4081=VERTEX_POINT ( 'NONE', #3177 ) ;
#4085=ORIENTED_EDGE ( 'NONE', *, *, #19157, .F. ) ;
#4087=EDGE_CURVE ( 'NONE', #10101, #19407, #9551, .T. ) ;
#4088=FACE_OUTER_BOUND ( 'NONE', #16266, .T. ) ;
#4089=DIRECTION ( 'NONE',  ( 0.000000000000000000, 1.000000000000000000, 0.000000000000000000 ) ) ;
#4092=DIRECTION ( 'NONE',  ( 1.000000000000000000, 0.000000000000000000, 0.000000000000000000 ) ) ;
#4099=AXIS2_PLACEMENT_3D ( 'NONE', #14136, #17270, #11114 ) ;
#4104=VERTEX_POINT ( 'NONE', #17817 ) ;
#4107=DIRECTION ( 'NONE',  ( 0.000000000000000000, -0.000000000000000000, 1.000000000000000000 ) ) ;
#4108=VERTEX_POINT ( 'NONE', #7979 ) ;
#4109=ORIENTED_EDGE ( 'NONE', *, *, #11312, .F. ) ;
#4112=EDGE_CURVE ( 'NONE', #4793, #15521, #15923, .T. ) ;
#4114=CARTESIAN_POINT ( 'NONE',  ( -7.626396343307448866, 0.000000000000000000, 0.000000000000000000 ) ) ;
#4115=EDGE_CURVE ( 'NONE', #13899, #8944, #6425, .T. ) ;
#4118=DIRECTION ( 'NONE',  ( 1.000000000000000000, 0.000000000000000000, 0.000000000000000000 ) ) ;
#4124=ORIENTED_EDGE ( 'NONE', *, *, #2849, .T. ) ;
#4126=DIRECTION ( 'NONE',  ( 1.000000000000000000, 0.000000000000000000, 0.000000000000000000 ) ) ;
#4133=ORIENTED_EDGE ( 'NONE', *, *, #11381, .F. ) ;
#4135=ORIENTED_EDGE ( 'NONE', *, *, #8761, .T. ) ;
#4137=EDGE_CURVE ( 'NONE', #3725, #7631, #1600, .T. ) ;
#4140=CYLINDRICAL_SURFACE ( 'NONE', #4331, 10.00000000000000000 ) ;
#4154=VERTEX_POINT ( 'NONE', #142 ) ;
#4157=EDGE_LOOP ( 'NONE', ( #19044, #9687, #1133, #18155 ) ) ;
#4158=DIRECTION ( 'NONE',  ( -0.000000000000000000, -0.000000000000000000, -1.000000000000000000 ) ) ;
#4161=EDGE_LOOP ( 'NONE', ( #2902, #3005, #20613, #16756 ) ) ;
#4163=EDGE_CURVE ( 'NONE', #6020, #19964, #19501, .T. ) ;
#4165=CARTESIAN_POINT ( 'NONE',  ( -17.94064177244175795, 11.64110105645932691, 10.00000000000000000 ) ) ;
#4166=DIRECTION ( 'NONE',  ( -0.000000000000000000, -0.000000000000000000, -1.000000000000000000 ) ) ;
#4174=ADVANCED_FACE ( 'NONE', ( #16342 ), #2017, .T. ) ;
#4178=DIRECTION ( 'NONE',  ( 0.000000000000000000, 1.000000000000000000, 0.000000000000000000 ) ) ;
#4181=LINE ( 'NONE', #10357, #11656 ) ;
#4186=SHAPE_REPRESENTATION_RELATIONSHIP ( 'NONE' , 'NONE' ,  #19662, #4314 ) ;
#4188=CARTESIAN_POINT ( 'NONE',  ( 30.00000000000000000, 10.00000000000000000, 1.000000000000000000 ) ) ;
#4205=ORIENTED_EDGE ( 'NONE', *, *, #4910, .F. ) ;
#4207=FACE_OUTER_BOUND ( 'NONE', #8278, .T. ) ;
#4208=ORIENTED_EDGE ( 'NONE', *, *, #13574, .F. ) ;
#4216=DIRECTION ( 'NONE',  ( 1.000000000000000000, 0.000000000000000000, 0.000000000000000000 ) ) ;
#4229=ORIENTED_EDGE ( 'NONE', *, *, #13976, .F. ) ;
#4231=DIRECTION ( 'NONE',  ( 0.000000000000000000, 0.000000000000000000, 1.000000000000000000 ) ) ;
#4233=VERTEX_POINT ( 'NONE', #7161 ) ;
#4237=EDGE_CURVE ( 'NONE', #11568, #16197, #5584, .T. ) ;
#4240=AXIS2_PLACEMENT_3D ( 'NONE', #2331, #13615, #10281 ) ;
#4241=ORIENTED_EDGE ( 'NONE', *, *, #3472, .F. ) ;
#4242=LINE ( 'NONE', #6021, #16007 ) ;
#4246=DIRECTION ( 'NONE',  ( -0.000000000000000000, 0.000000000000000000, -1.000000000000000000 ) ) ;
#4248=DIRECTION ( 'NONE',  ( -1.000000000000000000, 0.000000000000000000, 0.000000000000000000 ) ) ;
#4260=CARTESIAN_POINT ( 'NONE',  ( 0.000000000000000000, 11.64110105645932691, 10.00000000000000000 ) ) ;
#4263=ORIENTED_EDGE ( 'NONE', *, *, #16645, .T. ) ;
#4268=LINE ( 'NONE', #10868, #1291 ) ;
#4283=ORIENTED_EDGE ( 'NONE', *, *, #9109, .T. ) ;
#4291=VERTEX_POINT ( 'NONE', #5481 ) ;
#4292=EDGE_CURVE ( 'NONE', #17482, #2580, #13422, .T. ) ;
#4297=CARTESIAN_POINT ( 'NONE',  ( 30.00000000000000000, 10.00000000000000000, 0.000000000000000000 ) ) ;
#4311=DIRECTION ( 'NONE',  ( 0.000000000000000000, 0.000000000000000000, -1.000000000000000000 ) ) ;
#4314=ADVANCED_BREP_SHAPE_REPRESENTATION ( '', ( #18044, #18039 ), #5348 ) ;
#4315=DIRECTION ( 'NONE',  ( -0.000000000000000000, -0.000000000000000000, -1.000000000000000000 ) ) ;
#4326=DIRECTION ( 'NONE',  ( -1.000000000000000000, 0.000000000000000000, 0.000000000000000000 ) ) ;
#4331=AXIS2_PLACEMENT_3D ( 'NONE', #16893, #8948, #20157 ) ;
#4337=VERTEX_POINT ( 'NONE', #3909 ) ;
#4344=EDGE_LOOP ( 'NONE', ( #16836, #12333, #7819, #140 ) ) ;
#4347=ORIENTED_EDGE ( 'NONE', *, *, #10396, .F. ) ;
#4348=DIRECTION ( 'NONE',  ( 1.156482317317871331E-15, -1.000000000000000000, 0.000000000000000000 ) ) ;
#4355=VECTOR ( 'NONE', #2302, 1000.000000000000000 ) ;
#4357=PLANE ( 'NONE',  #6374 ) ;
#4362=VECTOR ( 'NONE', #18035, 1000.000000000000000 ) ;
#4364=ORIENTED_EDGE ( 'NONE', *, *, #949, .T. ) ;
#4367=ORIENTED_EDGE ( 'NONE', *, *, #2316, .T. ) ;
#4369=ORIENTED_EDGE ( 'NONE', *, *, #13574, .T. ) ;
#4374=DIRECTION ( 'NONE',  ( 0.000000000000000000, 1.000000000000000000, -0.000000000000000000 ) ) ;
#4389=ORIENTED_EDGE ( 'NONE', *, *, #5170, .F. ) ;
#4396=ORIENTED_EDGE ( 'NONE', *, *, #15117, .F. ) ;
#4400=DIRECTION ( 'NONE',  ( 0.000000000000000000, -1.000000000000000000, 0.000000000000000000 ) ) ;
#4403=AXIS2_PLACEMENT_3D ( 'NONE', #14938, #9165, #1323 ) ;
#4405=EDGE_CURVE ( 'NONE', #8442, #20408, #8424, .T. ) ;
#4410=CARTESIAN_POINT ( 'NONE',  ( 14.99999999999999645, 3.000000000000003553, 1.000000000000000000 ) ) ;
#4422=ORIENTED_EDGE ( 'NONE', *, *, #17515, .F. ) ;
#4423=DIRECTION ( 'NONE',  ( 1.000000000000000000, 0.000000000000000000, 0.000000000000000000 ) ) ;
#4427=ADVANCED_FACE ( 'NONE', ( #2860 ), #13622, .T. ) ;
#4430=VECTOR ( 'NONE', #359, 1000.000000000000000 ) ;
#4431=LINE ( 'NONE', #18454, #15397 ) ;
#4440=VECTOR ( 'NONE', #19791, 1000.000000000000000 ) ;
#4456=DIRECTION ( 'NONE',  ( 1.000000000000000000, -0.000000000000000000, -0.000000000000000000 ) ) ;
#4464=CARTESIAN_POINT ( 'NONE',  ( 0.000000000000000000, 10.00000000000000000, 1.000000000000000000 ) ) ;
#4465=DIRECTION ( 'NONE',  ( -1.000000000000000000, 0.000000000000000000, 0.000000000000000000 ) ) ;
#4471=EDGE_LOOP ( 'NONE', ( #9775, #13409, #18137, #6655 ) ) ;
#4473=DIRECTION ( 'NONE',  ( 1.000000000000000000, 0.000000000000000000, 0.000000000000000000 ) ) ;
#4476=VECTOR ( 'NONE', #1895, 1000.000000000000000 ) ;
#4480=PLANE ( 'NONE',  #10654 ) ;
#4481=CARTESIAN_POINT ( 'NONE',  ( -11.75209451496117197, 10.00000000000000000, 1.000000000000000000 ) ) ;
#4483=CARTESIAN_POINT ( 'NONE',  ( -10.38119784648305632, -14.00000000000000000, 2.000000000000000000 ) ) ;
#4490=CARTESIAN_POINT ( 'NONE',  ( 26.69203811574919882, 16.00000000000000000, 1.000000000000000000 ) ) ;
#4493=EDGE_CURVE ( 'NONE', #15313, #9004, #8407, .T. ) ;
#4495=LINE ( 'NONE', #15472, #20697 ) ;
#4496=VERTEX_POINT ( 'NONE', #18768 ) ;
#4501=CARTESIAN_POINT ( 'NONE',  ( -20.00349085826861995, 10.00000000000000000, 0.000000000000000000 ) ) ;
#4520=ORIENTED_EDGE ( 'NONE', *, *, #10684, .F. ) ;
#4524=VECTOR ( 'NONE', #5997, 1000.000000000000000 ) ;
#4529=CARTESIAN_POINT ( 'NONE',  ( -16.62779268661489951, 11.64110105645932691, 0.000000000000000000 ) ) ;
#4531=CARTESIAN_POINT ( 'NONE',  ( -5.381197846483055436, -6.000000000000000000, 2.000000000000000000 ) ) ;
#4535=ORIENTED_EDGE ( 'NONE', *, *, #2638, .F. ) ;
#4537=DIRECTION ( 'NONE',  ( -0.000000000000000000, 0.000000000000000000, -1.000000000000000000 ) ) ;
#4545=VECTOR ( 'NONE', #17648, 1000.000000000000000 ) ;
#4551=CARTESIAN_POINT ( 'NONE',  ( 14.31494360078803041, 0.000000000000000000, 1.000000000000000000 ) ) ;
#4558=DIRECTION ( 'NONE',  ( -1.000000000000000000, 0.000000000000000000, 0.000000000000000000 ) ) ;
#4566=ADVANCED_FACE ( 'NONE', ( #18457 ), #18658, .T. ) ;
#4568=DIRECTION ( 'NONE',  ( 0.000000000000000000, 0.000000000000000000, 1.000000000000000000 ) ) ;
#4569=ORIENTED_EDGE ( 'NONE', *, *, #3849, .F. ) ;
#4575=EDGE_CURVE ( 'NONE', #16197, #10885, #7671, .T. ) ;
#4576=CARTESIAN_POINT ( 'NONE',  ( -0.000000000000000000, 10.00000000000000000, 0.000000000000000000 ) ) ;
#4578=DIRECTION ( 'NONE',  ( -0.000000000000000000, 0.000000000000000000, -1.000000000000000000 ) ) ;
#4580=VECTOR ( 'NONE', #12544, 1000.000000000000000 ) ;
#4582=CARTESIAN_POINT ( 'NONE',  ( 15.06494360078803041, 0.000000000000000000, 1.000000000000000000 ) ) ;
#4591=CARTESIAN_POINT ( 'NONE',  ( -0.1250000000000001110, 16.00000000000000000, 1.000000000000000000 ) ) ;
#4593=DIRECTION ( 'NONE',  ( 0.000000000000000000, 0.000000000000000000, 1.000000000000000000 ) ) ;
#4600=ADVANCED_FACE ( 'NONE', ( #13932 ), #16973, .F. ) ;
#4613=ORIENTED_EDGE ( 'NONE', *, *, #11067, .T. ) ;
#4614=PRODUCT_DEFINITION_CONTEXT ( 'detailed design', #1200, 'design' ) ;
#4618=CLOSED_SHELL ( 'NONE', ( #14787, #4600, #3975, #6083, #20544, #1566, #12111, #12984, #16950, #8664, #4427, #15438, #4621, #13987, #1087, #20695, #14302, #4174, #17530, #13034, #20279, #15086, #6436, #1829, #16008, #4566, #10902, #36, #1103, #5264, #13456, #20399, #15396, #14857, #10042, #10284, #20268, #17488, #10143, #264, #8087, #14961, #9908, #8312, #16949, #20523, #10297, #3588, #5315, #12730, #4903, #9487, #4814, #20253, #2003, #16741, #15835, #12845, #6122, #9999, #12283, #1015, #12958, #13443, #3300, #7587, #14140, #920, #12803, #14253, #10904, #19991, #833, #9242, #3824, #5135, #3239, #2131, #17322, #3480, #12210, #11729, #6228, #18949, #19828, #16878, #3859, #11447, #6611, #12567, #16321, #10414, #18240, #461, #12671, #9031, #20120, #3151, #11174, #289, #19151, #5475, #14078, #9780, #11286, #9758, #20504, #18255, #7195, #8386, #897, #1197, #10043, #14094, #4896, #13030, #20616, #11313, #15289, #5935, #12284, #2309, #12427, #1240, #10941, #7909, #6464, #11463, #14587, #5743, #4787, #17462, #8597, #7569, #15408, #1471, #16110, #6550 ) ) ;
#4621=ADVANCED_FACE ( 'NONE', ( #18351 ), #5894, .T. ) ;
#4624=CARTESIAN_POINT ( 'NONE',  ( 22.56633994409548194, 10.00000000000000000, 1.000000000000000000 ) ) ;
#4634=CARTESIAN_POINT ( 'NONE',  ( -0.000000000000000000, 11.64110105645932691, 0.000000000000000000 ) ) ;
#4645=CARTESIAN_POINT ( 'NONE',  ( 0.000000000000000000, 10.00000000000000000, 1.000000000000000000 ) ) ;
#4646=ORIENTED_EDGE ( 'NONE', *, *, #10516, .F. ) ;
#4650=VECTOR ( 'NONE', #19637, 1000.000000000000000 ) ;
#4665=ORIENTED_EDGE ( 'NONE', *, *, #9662, .T. ) ;
#4667=PLANE ( 'NONE',  #6 ) ;
#4668=VERTEX_POINT ( 'NONE', #19185 ) ;
#4669=EDGE_CURVE ( 'NONE', #7911, #7740, #1807, .T. ) ;
#4670=PLANE ( 'NONE',  #2964 ) ;
#4671=ORIENTED_EDGE ( 'NONE', *, *, #14597, .F. ) ;
#4673=VECTOR ( 'NONE', #12670, 1000.000000000000000 ) ;
#4674=ORIENTED_EDGE ( 'NONE', *, *, #7490, .T. ) ;
#4685=DIRECTION ( 'NONE',  ( -0.000000000000000000, -0.000000000000000000, -1.000000000000000000 ) ) ;
#4688=ORIENTED_EDGE ( 'NONE', *, *, #1, .T. ) ;
#4690=DIRECTION ( 'NONE',  ( 0.000000000000000000, 0.000000000000000000, 1.000000000000000000 ) ) ;
#4699=VERTEX_POINT ( 'NONE', #17278 ) ;
#4701=ORIENTED_EDGE ( 'NONE', *, *, #17294, .T. ) ;
#4723=ORIENTED_EDGE ( 'NONE', *, *, #15494, .F. ) ;
#4726=LINE ( 'NONE', #222, #1108 ) ;
#4730=DIRECTION ( 'NONE',  ( 0.000000000000000000, -0.000000000000000000, 1.000000000000000000 ) ) ;
#4734=DIRECTION ( 'NONE',  ( 0.000000000000000000, 1.000000000000000000, 0.000000000000000000 ) ) ;
#4741=DIRECTION ( 'NONE',  ( 0.000000000000000000, -1.000000000000000000, 0.000000000000000000 ) ) ;
#4744=ORIENTED_EDGE ( 'NONE', *, *, #13240, .F. ) ;
#4747=DIRECTION ( 'NONE',  ( 1.000000000000000000, 0.000000000000000000, 0.000000000000000000 ) ) ;
#4752=VECTOR ( 'NONE', #15843, 1000.000000000000000 ) ;
#4756=DIRECTION ( 'NONE',  ( 1.000000000000000000, 0.000000000000000000, 0.000000000000000000 ) ) ;
#4758=PLANE ( 'NONE',  #639 ) ;
#4761=FACE_OUTER_BOUND ( 'NONE', #14309, .T. ) ;
#4762=LINE ( 'NONE', #11147, #3352 ) ;
#4778=ORIENTED_EDGE ( 'NONE', *, *, #3127, .F. ) ;
#4779=CARTESIAN_POINT ( 'NONE',  ( 19.19064177244175440, 10.00000000000000000, 0.000000000000000000 ) ) ;
#4782=AXIS2_PLACEMENT_3D ( 'NONE', #6172, #4593, #19046 ) ;
#4783=DIRECTION ( 'NONE',  ( 0.000000000000000000, -0.000000000000000000, 1.000000000000000000 ) ) ;
#4785=PLANE ( 'NONE',  #18004 ) ;
#4787=ADVANCED_FACE ( 'NONE', ( #9755 ), #16140, .F. ) ;
#4792=VECTOR ( 'NONE', #7210, 1000.000000000000000 ) ;
#4793=VERTEX_POINT ( 'NONE', #14144 ) ;
#4800=EDGE_CURVE ( 'NONE', #9362, #6964, #20551, .T. ) ;
#4801=CARTESIAN_POINT ( 'NONE',  ( 20.50349085826861995, 10.00000000000000000, 0.000000000000000000 ) ) ;
#4803=ORIENTED_EDGE ( 'NONE', *, *, #2928, .T. ) ;
#4807=EDGE_CURVE ( 'NONE', #16861, #13083, #7877, .T. ) ;
#4809=VERTEX_POINT ( 'NONE', #31 ) ;
#4814=ADVANCED_FACE ( 'NONE', ( #6302 ), #343, .T. ) ;
#4828=EDGE_LOOP ( 'NONE', ( #7771, #1102, #3440, #16016 ) ) ;
#4829=EDGE_LOOP ( 'NONE', ( #18627, #11636, #8292, #1819 ) ) ;
#4835=EDGE_CURVE ( 'NONE', #2170, #13899, #5049, .T. ) ;
#4842=ORIENTED_EDGE ( 'NONE', *, *, #18197, .F. ) ;
#4852=ORIENTED_EDGE ( 'NONE', *, *, #409, .F. ) ;
#4855=CARTESIAN_POINT ( 'NONE',  ( 15.00000000000000000, 0.000000000000000000, 1.000000000000000000 ) ) ;
#4859=DIRECTION ( 'NONE',  ( 1.000000000000000000, 0.000000000000000000, -0.000000000000000000 ) ) ;
#4877=CARTESIAN_POINT ( 'NONE',  ( 0.000000000000000000, 16.00000000000000000, 1.000000000000000000 ) ) ;
#4880=ORIENTED_EDGE ( 'NONE', *, *, #2536, .T. ) ;
#4882=DIRECTION ( 'NONE',  ( -0.000000000000000000, -0.000000000000000000, -1.000000000000000000 ) ) ;
#4888=CARTESIAN_POINT ( 'NONE',  ( -15.87779268661489773, 10.00000000000000000, 0.000000000000000000 ) ) ;
#4895=ORIENTED_EDGE ( 'NONE', *, *, #9073, .F. ) ;
#4896=ADVANCED_FACE ( 'NONE', ( #18125 ), #446, .T. ) ;
#4897=FACE_OUTER_BOUND ( 'NONE', #7017, .T. ) ;
#4900=CARTESIAN_POINT ( 'NONE',  ( -5.563547257480587760, 10.00000000000000000, 1.000000000000000000 ) ) ;
#4903=ADVANCED_FACE ( 'NONE', ( #6825 ), #8703, .T. ) ;
#4910=EDGE_CURVE ( 'NONE', #2930, #3253, #6619, .T. ) ;
#4913=DIRECTION ( 'NONE',  ( -0.000000000000000000, -1.000000000000000000, -0.000000000000000000 ) ) ;
#4917=CARTESIAN_POINT ( 'NONE',  ( 27.00000000000000000, 3.000000000000000000, 1.000000000000000000 ) ) ;
#4937=CARTESIAN_POINT ( 'NONE',  ( -27.94203811574922725, 3.231447299068595019E-14, 0.000000000000000000 ) ) ;
#4943=ORIENTED_EDGE ( 'NONE', *, *, #14069, .T. ) ;
#4946=AXIS2_PLACEMENT_3D ( 'NONE', #11382, #11683, #3748 ) ;
#4955=ORIENTED_EDGE ( 'NONE', *, *, #5239, .T. ) ;
#4959=( GEOMETRIC_REPRESENTATION_CONTEXT ( 3 ) GLOBAL_UNCERTAINTY_ASSIGNED_CONTEXT ( ( #8824 ) ) GLOBAL_UNIT_ASSIGNED_CONTEXT ( ( #16287, #13147, #5198 ) ) REPRESENTATION_CONTEXT ( 'NONE', 'WORKASPACE' ) );
#4960=LINE ( 'NONE', #8307, #12311 ) ;
#4967=CARTESIAN_POINT ( 'NONE',  ( 15.06494360078803041, 10.00000000000000000, 1.000000000000000000 ) ) ;
#4977=CARTESIAN_POINT ( 'NONE',  ( -16.62779268661489951, 0.000000000000000000, 0.000000000000000000 ) ) ;
#4982=CARTESIAN_POINT ( 'NONE',  ( 24.62918902992234038, 11.64110105645932691, 0.000000000000000000 ) ) ;
#4992=EDGE_CURVE ( 'NONE', #14620, #4337, #19692, .T. ) ;
#4996=VERTEX_POINT ( 'NONE', #18434 ) ;
#5001=CARTESIAN_POINT ( 'NONE',  ( 21.25349085826861995, 10.00000000000000000, 1.000000000000000000 ) ) ;
#5003=VECTOR ( 'NONE', #14156, 1000.000000000000000 ) ;
#5008=VECTOR ( 'NONE', #7644, 1000.000000000000000 ) ;
#5016=EDGE_CURVE ( 'NONE', #12491, #8181, #2625, .T. ) ;
#5023=VECTOR ( 'NONE', #13696, 1000.000000000000000 ) ;
#5024=PLANE ( 'NONE',  #3706 ) ;
#5032=CARTESIAN_POINT ( 'NONE',  ( -15.00000000000000000, -6.000000000000000000, 1.000000000000000000 ) ) ;
#5033=EDGE_LOOP ( 'NONE', ( #15136, #18546, #3025, #7583 ) ) ;
#5037=CYLINDRICAL_SURFACE ( 'NONE', #4099, 10.00000000000000000 ) ;
#5039=CARTESIAN_POINT ( 'NONE',  ( -22.06633994409548194, 11.64110105645932691, 10.00000000000000000 ) ) ;
#5040=VECTOR ( 'NONE', #16476, 1000.000000000000000 ) ;
#5041=AXIS2_PLACEMENT_3D ( 'NONE', #20165, #17111, #2793 ) ;
#5049=LINE ( 'NONE', #16339, #17070 ) ;
#5055=DIRECTION ( 'NONE',  ( 1.000000000000000000, 0.000000000000000000, 0.000000000000000000 ) ) ;
#5062=PLANE ( 'NONE',  #12667 ) ;
#5064=EDGE_CURVE ( 'NONE', #7837, #965, #1169, .T. ) ;
#5065=EDGE_LOOP ( 'NONE', ( #19511, #11358, #4124, #12971 ) ) ;
#5080=EDGE_LOOP ( 'NONE', ( #10676, #5283, #16588, #4520 ) ) ;
#5086=CARTESIAN_POINT ( 'NONE',  ( -7.500000000000000888, -9.999999999999992895, 2.000000000000000000 ) ) ;
#5087=ORIENTED_EDGE ( 'NONE', *, *, #16692, .F. ) ;
#5088=ORIENTED_EDGE ( 'NONE', *, *, #197, .F. ) ;
#5089=AXIS2_PLACEMENT_3D ( 'NONE', #11062, #15958, #19536 ) ;
#5092=CARTESIAN_POINT ( 'NONE',  ( 0.000000000000000000, 10.00000000000000000, 1.000000000000000000 ) ) ;
#5093=VERTEX_POINT ( 'NONE', #17368 ) ;
#5116=CARTESIAN_POINT ( 'NONE',  ( -20.00349085826861995, 10.00000000000000000, 1.000000000000000000 ) ) ;
#5134=ORIENTED_EDGE ( 'NONE', *, *, #18812, .F. ) ;
#5135=ADVANCED_FACE ( 'NONE', ( #2095 ), #8479, .T. ) ;
#5137=EDGE_CURVE ( 'NONE', #2654, #20035, #3867, .T. ) ;
#5139=FACE_OUTER_BOUND ( 'NONE', #5080, .T. ) ;
#5146=LINE ( 'NONE', #11620, #7062 ) ;
#5154=CARTESIAN_POINT ( 'NONE',  ( 0.000000000000000000, 10.00000000000000000, 1.000000000000000000 ) ) ;
#5162=VERTEX_POINT ( 'NONE', #14637 ) ;
#5163=LINE ( 'NONE', #14679, #9119 ) ;
#5166=LINE ( 'NONE', #3703, #10335 ) ;
#5168=CARTESIAN_POINT ( 'NONE',  ( -20.75349085826862350, 0.000000000000000000, 1.000000000000000000 ) ) ;
#5170=EDGE_CURVE ( 'NONE', #18231, #14087, #1889, .T. ) ;
#5174=EDGE_CURVE ( 'NONE', #20463, #2481, #16316, .T. ) ;
#5186=ORIENTED_EDGE ( 'NONE', *, *, #13582, .F. ) ;
#5188=ORIENTED_EDGE ( 'NONE', *, *, #356, .T. ) ;
#5189=DIRECTION ( 'NONE',  ( 1.000000000000000000, 0.000000000000000000, 0.000000000000000000 ) ) ;
#5191=ORIENTED_EDGE ( 'NONE', *, *, #118, .F. ) ;
#5196=DIRECTION ( 'NONE',  ( 0.000000000000000000, -0.000000000000000000, 1.000000000000000000 ) ) ;
#5198=( NAMED_UNIT ( * ) SI_UNIT ( $, .STERADIAN. ) SOLID_ANGLE_UNIT ( ) );
#5201=CARTESIAN_POINT ( 'NONE',  ( -26.19203811574920593, 10.00000000000000000, 0.000000000000000000 ) ) ;
#5214=ORIENTED_EDGE ( 'NONE', *, *, #8761, .F. ) ;
#5215=CARTESIAN_POINT ( 'NONE',  ( 9.000000000000000000, -9.999999999999991118, 2.000000000000000000 ) ) ;
#5234=( LENGTH_UNIT ( ) NAMED_UNIT ( * ) SI_UNIT ( .MILLI., .METRE. ) );
#5239=EDGE_CURVE ( 'NONE', #15313, #886, #16220, .T. ) ;
#5241=LINE ( 'NONE', #17903, #508 ) ;
#5250=VECTOR ( 'NONE', #17358, 1000.000000000000000 ) ;
#5253=ORIENTED_EDGE ( 'NONE', *, *, #20182, .F. ) ;
#5263=CARTESIAN_POINT ( 'NONE',  ( 15.00000000000000355, -5.999999999999996447, 2.000000000000000000 ) ) ;
#5264=ADVANCED_FACE ( 'NONE', ( #6902 ), #3768, .T. ) ;
#5268=EDGE_CURVE ( 'NONE', #18649, #15262, #19669, .T. ) ;
#5273=CARTESIAN_POINT ( 'NONE',  ( 29.71062960567705602, 11.64110105645932691, 0.000000000000000000 ) ) ;
#5276=EDGE_LOOP ( 'NONE', ( #20683, #14495, #20184, #17727 ) ) ;
#5280=ORIENTED_EDGE ( 'NONE', *, *, #17117, .F. ) ;
#5283=ORIENTED_EDGE ( 'NONE', *, *, #8211, .T. ) ;
#5291=DIRECTION ( 'NONE',  ( 0.000000000000000000, 0.000000000000000000, 1.000000000000000000 ) ) ;
#5293=VECTOR ( 'NONE', #1085, 1000.000000000000000 ) ;
#5296=VECTOR ( 'NONE', #7060, 1000.000000000000000 ) ;
#5297=DIRECTION ( 'NONE',  ( -5.782411586589356653E-16, 1.000000000000000000, -0.000000000000000000 ) ) ;
#5301=EDGE_CURVE ( 'NONE', #5810, #16102, #13174, .T. ) ;
#5309=LINE ( 'NONE', #10021, #13006 ) ;
#5310=ORIENTED_EDGE ( 'NONE', *, *, #17168, .F. ) ;
#5311=VECTOR ( 'NONE', #12117, 1000.000000000000000 ) ;
#5312=AXIS2_PLACEMENT_3D ( 'NONE', #12370, #1089, #12163 ) ;
#5314=ORIENTED_EDGE ( 'NONE', *, *, #1849, .F. ) ;
#5315=ADVANCED_FACE ( 'NONE', ( #11509 ), #8377, .T. ) ;
#5319=VECTOR ( 'NONE', #586, 1000.000000000000000 ) ;
#5321=CARTESIAN_POINT ( 'NONE',  ( -0.000000000000000000, 0.000000000000000000, 0.000000000000000000 ) ) ;
#5323=LINE ( 'NONE', #16134, #5679 ) ;
#5330=EDGE_CURVE ( 'NONE', #9626, #6206, #9937, .T. ) ;
#5332=AXIS2_PLACEMENT_3D ( 'NONE', #18395, #10443, #2480 ) ;
#5334=CARTESIAN_POINT ( 'NONE',  ( 0.000000000000000000, 16.00000000000000000, 1.000000000000000000 ) ) ;
#5341=FACE_OUTER_BOUND ( 'NONE', #3281, .T. ) ;
#5342=CARTESIAN_POINT ( 'NONE',  ( -26.94203811574920593, 11.64110105645932691, 10.00000000000000000 ) ) ;
#5348=( GEOMETRIC_REPRESENTATION_CONTEXT ( 3 ) GLOBAL_UNCERTAINTY_ASSIGNED_CONTEXT ( ( #3518 ) ) GLOBAL_UNIT_ASSIGNED_CONTEXT ( ( #13277, #13183, #9842 ) ) REPRESENTATION_CONTEXT ( 'NONE', 'WORKASPACE' ) );
#5362=ORIENTED_EDGE ( 'NONE', *, *, #3743, .F. ) ;
#5365=FACE_OUTER_BOUND ( 'NONE', #8801, .T. ) ;
#5369=ORIENTED_EDGE ( 'NONE', *, *, #14037, .T. ) ;
#5373=LINE ( 'NONE', #11643, #8317 ) ;
#5376=CARTESIAN_POINT ( 'NONE',  ( 6.063547257480584207, 11.64110105645932691, 10.00000000000000000 ) ) ;
#5377=CARTESIAN_POINT ( 'NONE',  ( 13.00209451496117374, 0.000000000000000000, 1.000000000000000000 ) ) ;
#5380=CARTESIAN_POINT ( 'NONE',  ( -9.689245429134309973, 11.64110105645932691, 10.00000000000000000 ) ) ;
#5391=CARTESIAN_POINT ( 'NONE',  ( -10.49999999999999822, -9.999999999999992895, 1.000000000000000000 ) ) ;
#5393=ORIENTED_EDGE ( 'NONE', *, *, #2849, .F. ) ;
#5403=DIRECTION ( 'NONE',  ( 0.000000000000000000, 1.000000000000000000, -0.000000000000000000 ) ) ;
#5407=DIRECTION ( 'NONE',  ( 0.000000000000000000, -1.000000000000000000, 0.000000000000000000 ) ) ;
#5411=AXIS2_PLACEMENT_3D ( 'NONE', #2191, #7011, #15053 ) ;
#5419=DIRECTION ( 'NONE',  ( -0.000000000000000000, -0.000000000000000000, -1.000000000000000000 ) ) ;
#5420=VERTEX_POINT ( 'NONE', #2716 ) ;
#5423=ORIENTED_EDGE ( 'NONE', *, *, #27, .F. ) ;
#5427=DIRECTION ( 'NONE',  ( 0.000000000000000000, 0.000000000000000000, -1.000000000000000000 ) ) ;
#5428=CIRCLE ( 'NONE', #2084, 1.499999999999998668 ) ;
#5432=DIRECTION ( 'NONE',  ( 1.000000000000000000, 0.000000000000000000, 0.000000000000000000 ) ) ;
#5434=DIRECTION ( 'NONE',  ( 0.000000000000000000, 0.000000000000000000, -1.000000000000000000 ) ) ;
#5439=EDGE_LOOP ( 'NONE', ( #16761, #12416, #8916, #5568 ) ) ;
#5452=PLANE ( 'NONE',  #3030 ) ;
#5453=EDGE_CURVE ( 'NONE', #13535, #3666, #16727, .T. ) ;
#5473=ORIENTED_EDGE ( 'NONE', *, *, #17937, .F. ) ;
#5475=ADVANCED_FACE ( 'NONE', ( #18301 ), #9096, .T. ) ;
#5476=LINE ( 'NONE', #16354, #17254 ) ;
#5477=DIRECTION ( 'NONE',  ( 1.000000000000000000, -0.000000000000000000, 0.000000000000000000 ) ) ;
#5478=FACE_OUTER_BOUND ( 'NONE', #5033, .T. ) ;
#5480=DIRECTION ( 'NONE',  ( 0.000000000000000000, 0.000000000000000000, -1.000000000000000000 ) ) ;
#5481=CARTESIAN_POINT ( 'NONE',  ( -24.87918902992234393, 10.00000000000000000, 1.000000000000000000 ) ) ;
#5483=LINE ( 'NONE', #16560, #6654 ) ;
#5495=DIRECTION ( 'NONE',  ( 0.000000000000000000, 1.000000000000000000, -0.000000000000000000 ) ) ;
#5499=CARTESIAN_POINT ( 'NONE',  ( 8.126396343307449754, 0.000000000000000000, 1.000000000000000000 ) ) ;
#5506=CARTESIAN_POINT ( 'NONE',  ( -2.187849085826861550, 11.64110105645932691, 10.00000000000000000 ) ) ;
#5507=EDGE_CURVE ( 'NONE', #7382, #12312, #15568, .T. ) ;
#5509=EDGE_CURVE ( 'NONE', #18680, #8532, #7218, .T. ) ;
#5517=ORIENTED_EDGE ( 'NONE', *, *, #5913, .F. ) ;
#5518=VECTOR ( 'NONE', #1321, 1000.000000000000000 ) ;
#5522=ORIENTED_EDGE ( 'NONE', *, *, #7932, .F. ) ;
#5523=EDGE_LOOP ( 'NONE', ( #20073, #2123, #15205, #11767 ) ) ;
#5524=AXIS2_PLACEMENT_3D ( 'NONE', #4582, #6366, #1351 ) ;
#5535=EDGE_CURVE ( 'NONE', #4699, #4291, #15363, .T. ) ;
#5540=DIRECTION ( 'NONE',  ( -1.000000000000000000, 0.000000000000000000, 0.000000000000000000 ) ) ;
#5545=VERTEX_POINT ( 'NONE', #5755 ) ;
#5568=ORIENTED_EDGE ( 'NONE', *, *, #7869, .F. ) ;
#5571=DIRECTION ( 'NONE',  ( 1.000000000000000000, -0.000000000000000000, 0.000000000000000000 ) ) ;
#5572=ORIENTED_EDGE ( 'NONE', *, *, #14394, .F. ) ;
#5575=VECTOR ( 'NONE', #6250, 1000.000000000000000 ) ;
#5577=EDGE_CURVE ( 'NONE', #12312, #2482, #13993, .T. ) ;
#5579=CARTESIAN_POINT ( 'NONE',  ( 21.25349085826861995, 16.00000000000000000, 1.000000000000000000 ) ) ;
#5580=DIRECTION ( 'NONE',  ( 0.000000000000000000, 1.000000000000000000, -0.000000000000000000 ) ) ;
#5584=LINE ( 'NONE', #19927, #13718 ) ;
#5589=ORIENTED_EDGE ( 'NONE', *, *, #11713, .T. ) ;
#5592=EDGE_CURVE ( 'NONE', #15085, #13339, #3396, .T. ) ;
#5604=CARTESIAN_POINT ( 'NONE',  ( -12.50209451496117197, 16.00000000000000000, 1.000000000000000000 ) ) ;
#5605=AXIS2_PLACEMENT_3D ( 'NONE', #7527, #5540, #13483 ) ;
#5611=DIRECTION ( 'NONE',  ( 0.000000000000000000, 0.000000000000000000, 1.000000000000000000 ) ) ;
#5622=AXIS2_PLACEMENT_3D ( 'NONE', #10127, #6787, #13054 ) ;
#5624=CARTESIAN_POINT ( 'NONE',  ( -20.00349085826861995, 16.00000000000000000, 1.000000000000000000 ) ) ;
#5625=CARTESIAN_POINT ( 'NONE',  ( 12.25209451496117197, 10.00000000000000000, 1.000000000000000000 ) ) ;
#5628=EDGE_LOOP ( 'NONE', ( #8691, #710, #13444, #13775 ) ) ;
#5633=DIRECTION ( 'NONE',  ( -0.000000000000000000, -0.000000000000000000, -1.000000000000000000 ) ) ;
#5643=DIRECTION ( 'NONE',  ( 0.000000000000000000, 0.000000000000000000, -1.000000000000000000 ) ) ;
#5650=ORIENTED_EDGE ( 'NONE', *, *, #19626, .F. ) ;
#5660=DIRECTION ( 'NONE',  ( 1.000000000000000000, 0.000000000000000000, 0.000000000000000000 ) ) ;
#5662=CIRCLE ( 'NONE', #17346, 2.999999999999999112 ) ;
#5665=AXIS2_PLACEMENT_3D ( 'NONE', #7460, #7152, #4107 ) ;
#5668=DIRECTION ( 'NONE',  ( 0.000000000000000000, -1.000000000000000000, 0.000000000000000000 ) ) ;
#5673=EDGE_CURVE ( 'NONE', #18307, #18399, #17451, .T. ) ;
#5679=VECTOR ( 'NONE', #9540, 1000.000000000000000 ) ;
#5683=CARTESIAN_POINT ( 'NONE',  ( -0.000000000000000000, 10.00000000000000000, 0.000000000000000000 ) ) ;
#5684=VECTOR ( 'NONE', #18511, 1000.000000000000000 ) ;
#5686=CARTESIAN_POINT ( 'NONE',  ( -24.87918902992234393, 10.00000000000000000, 0.000000000000000000 ) ) ;
#5687=EDGE_CURVE ( 'NONE', #14757, #15085, #15671, .T. ) ;
#5704=ORIENTED_EDGE ( 'NONE', *, *, #18453, .F. ) ;
#5707=DIRECTION ( 'NONE',  ( -1.156482317317871133E-15, -1.000000000000000000, 0.000000000000000000 ) ) ;
#5710=DIRECTION ( 'NONE',  ( 0.000000000000000000, -1.000000000000000000, 0.000000000000000000 ) ) ;
#5713=ORIENTED_EDGE ( 'NONE', *, *, #11261, .F. ) ;
#5717=FACE_OUTER_BOUND ( 'NONE', #15828, .T. ) ;
#5720=DIRECTION ( 'NONE',  ( 0.000000000000000000, -1.000000000000000000, 0.000000000000000000 ) ) ;
#5726=DIRECTION ( 'NONE',  ( 0.000000000000000000, 0.000000000000000000, 1.000000000000000000 ) ) ;
#5732=VERTEX_POINT ( 'NONE', #4490 ) ;
#5738=CARTESIAN_POINT ( 'NONE',  ( -15.87779268661489773, 0.000000000000000000, 1.000000000000000000 ) ) ;
#5743=ADVANCED_FACE ( 'NONE', ( #1658 ), #6256, .F. ) ;
#5749=CARTESIAN_POINT ( 'NONE',  ( 1.937849085826861328, 10.00000000000000000, 1.000000000000000000 ) ) ;
#5753=ORIENTED_EDGE ( 'NONE', *, *, #13835, .T. ) ;
#5755=CARTESIAN_POINT ( 'NONE',  ( -17.94064177244175795, 11.64110105645932691, 0.000000000000000000 ) ) ;
#5762=CARTESIAN_POINT ( 'NONE',  ( -10.38119784648305632, -14.00000000000000000, 2.000000000000000000 ) ) ;
#5764=AXIS2_PLACEMENT_3D ( 'NONE', #6543, #7901, #11047 ) ;
#5765=CARTESIAN_POINT ( 'NONE',  ( 15.00000000000000355, -5.999999999999996447, 2.000000000000000000 ) ) ;
#5769=CARTESIAN_POINT ( 'NONE',  ( -7.500000000000000888, -9.999999999999992895, 2.000000000000000000 ) ) ;
#5772=LINE ( 'NONE', #952, #15728 ) ;
#5777=FACE_OUTER_BOUND ( 'NONE', #15242, .T. ) ;
#5779=EDGE_CURVE ( 'NONE', #16197, #20119, #13406, .T. ) ;
#5785=ORIENTED_EDGE ( 'NONE', *, *, #8063, .T. ) ;
#5786=ORIENTED_EDGE ( 'NONE', *, *, #13749, .T. ) ;
#5794=DIRECTION ( 'NONE',  ( 1.000000000000000000, 0.000000000000000000, 0.000000000000000000 ) ) ;
#5796=DIRECTION ( 'NONE',  ( 0.000000000000000000, -0.000000000000000000, 1.000000000000000000 ) ) ;
#5800=ORIENTED_EDGE ( 'NONE', *, *, #11830, .F. ) ;
#5810=VERTEX_POINT ( 'NONE', #18898 ) ;
#5811=DIRECTION ( 'NONE',  ( 0.000000000000000000, 1.000000000000000000, -0.000000000000000000 ) ) ;
#5825=DIRECTION ( 'NONE',  ( -0.000000000000000000, -0.000000000000000000, -1.000000000000000000 ) ) ;
#5827=CARTESIAN_POINT ( 'NONE',  ( 4.750698171653723989, 10.00000000000000000, 0.000000000000000000 ) ) ;
#5835=ORIENTED_EDGE ( 'NONE', *, *, #4163, .T. ) ;
#5836=EDGE_CURVE ( 'NONE', #15932, #8657, #8673, .T. ) ;
#5837=LINE ( 'NONE', #17015, #18317 ) ;
#5841=ORIENTED_EDGE ( 'NONE', *, *, #15509, .T. ) ;
#5843=CARTESIAN_POINT ( 'NONE',  ( 4.750698171653723989, 0.000000000000000000, 1.000000000000000000 ) ) ;
#5850=CARTESIAN_POINT ( 'NONE',  ( 25.37918902992234393, 16.00000000000000000, 1.000000000000000000 ) ) ;
#5861=ORIENTED_EDGE ( 'NONE', *, *, #14349, .T. ) ;
#5866=DIRECTION ( 'NONE',  ( -0.4999999999999947264, -0.8660254037844417052, 0.000000000000000000 ) ) ;
#5877=CARTESIAN_POINT ( 'NONE',  ( 0.000000000000000000, 11.64110105645932691, 10.00000000000000000 ) ) ;
#5884=ORIENTED_EDGE ( 'NONE', *, *, #14507, .T. ) ;
#5894=PLANE ( 'NONE',  #18096 ) ;
#5909=EDGE_CURVE ( 'NONE', #18372, #18307, #13418, .T. ) ;
#5913=EDGE_CURVE ( 'NONE', #20101, #12443, #13014, .T. ) ;
#5917=CARTESIAN_POINT ( 'NONE',  ( 23.31633994409548549, 10.00000000000000000, 1.000000000000000000 ) ) ;
#5920=CARTESIAN_POINT ( 'NONE',  ( 0.000000000000000000, 10.00000000000000000, 1.000000000000000000 ) ) ;
#5922=DIRECTION ( 'NONE',  ( -0.000000000000000000, -0.000000000000000000, -1.000000000000000000 ) ) ;
#5929=VERTEX_POINT ( 'NONE', #3400 ) ;
#5933=VECTOR ( 'NONE', #24, 1000.000000000000000 ) ;
#5934=DIRECTION ( 'NONE',  ( -0.000000000000000000, -0.000000000000000000, -1.000000000000000000 ) ) ;
#5935=ADVANCED_FACE ( 'NONE', ( #4761 ), #17421, .T. ) ;
#5939=LINE ( 'NONE', #13669, #20356 ) ;
#5940=DIRECTION ( 'NONE',  ( 0.000000000000000000, 1.000000000000000000, -0.000000000000000000 ) ) ;
#5942=FACE_OUTER_BOUND ( 'NONE', #16393, .T. ) ;
#5949=ORIENTED_EDGE ( 'NONE', *, *, #9322, .T. ) ;
#5953=VERTEX_POINT ( 'NONE', #15743 ) ;
#5957=VERTEX_POINT ( 'NONE', #12809 ) ;
#5958=EDGE_CURVE ( 'NONE', #932, #19920, #9472, .T. ) ;
#5974=VECTOR ( 'NONE', #12160, 1000.000000000000000 ) ;
#5990=VECTOR ( 'NONE', #489, 1000.000000000000000 ) ;
#5995=EDGE_CURVE ( 'NONE', #15113, #14620, #14436, .T. ) ;
#5996=CYLINDRICAL_SURFACE ( 'NONE', #5312, 10.00000000000000000 ) ;
#5997=DIRECTION ( 'NONE',  ( 0.000000000000000000, -1.000000000000000000, 0.000000000000000000 ) ) ;
#5998=CARTESIAN_POINT ( 'NONE',  ( 5.381197846483058989, -14.00000000000000000, 2.000000000000000000 ) ) ;
#5999=DIRECTION ( 'NONE',  ( 0.000000000000000000, 0.000000000000000000, 1.000000000000000000 ) ) ;
#6008=VECTOR ( 'NONE', #4747, 1000.000000000000000 ) ;
#6018=DIRECTION ( 'NONE',  ( 0.000000000000000000, 1.000000000000000000, 0.000000000000000000 ) ) ;
#6019=DIRECTION ( 'NONE',  ( 1.000000000000000000, 0.000000000000000000, 0.000000000000000000 ) ) ;
#6020=VERTEX_POINT ( 'NONE', #7806 ) ;
#6021=CARTESIAN_POINT ( 'NONE',  ( 10.38119784648305810, -14.00000000000000000, 1.000000000000000000 ) ) ;
#6024=VECTOR ( 'NONE', #19484, 1000.000000000000000 ) ;
#6029=VECTOR ( 'NONE', #777, 1000.000000000000000 ) ;
#6030=EDGE_CURVE ( 'NONE', #15705, #175, #12905, .T. ) ;
#6031=DIRECTION ( 'NONE',  ( 1.000000000000000000, -0.000000000000000000, 0.000000000000000000 ) ) ;
#6033=CARTESIAN_POINT ( 'NONE',  ( 27.94203811574922725, 3.231447299068595019E-14, 1.000000000000000000 ) ) ;
#6038=VERTEX_POINT ( 'NONE', #16166 ) ;
#6041=DIRECTION ( 'NONE',  ( 0.000000000000000000, 0.000000000000000000, -1.000000000000000000 ) ) ;
#6044=FACE_OUTER_BOUND ( 'NONE', #1210, .T. ) ;
#6046=ORIENTED_EDGE ( 'NONE', *, *, #1849, .T. ) ;
#6049=AXIS2_PLACEMENT_3D ( 'NONE', #15825, #9652, #17712 ) ;
#6074=ORIENTED_EDGE ( 'NONE', *, *, #10792, .F. ) ;
#6079=VECTOR ( 'NONE', #17889, 1000.000000000000000 ) ;
#6080=CARTESIAN_POINT ( 'NONE',  ( -5.381197846483055436, -14.00000000000000000, 2.000000000000000000 ) ) ;
#6083=ADVANCED_FACE ( 'NONE', ( #9672 ), #12704, .T. ) ;
#6084=EDGE_CURVE ( 'NONE', #20035, #6794, #12923, .T. ) ;
#6085=CARTESIAN_POINT ( 'NONE',  ( 16.37779268661489596, 10.00000000000000000, 1.000000000000000000 ) ) ;
#6094=ORIENTED_EDGE ( 'NONE', *, *, #18843, .F. ) ;
#6098=ORIENTED_EDGE ( 'NONE', *, *, #14680, .T. ) ;
#6106=DIRECTION ( 'NONE',  ( 0.000000000000000000, -1.000000000000000000, 0.000000000000000000 ) ) ;
#6108=CARTESIAN_POINT ( 'NONE',  ( -20.00349085826861995, 10.00000000000000000, 1.000000000000000000 ) ) ;
#6111=ORIENTED_EDGE ( 'NONE', *, *, #2536, .F. ) ;
#6116=VERTEX_POINT ( 'NONE', #4982 ) ;
#6118=CARTESIAN_POINT ( 'NONE',  ( -18.69064177244175795, 10.00000000000000000, 1.000000000000000000 ) ) ;
#6119=EDGE_LOOP ( 'NONE', ( #4229, #2375, #18773, #17453 ) ) ;
#6120=ORIENTED_EDGE ( 'NONE', *, *, #16252, .T. ) ;
#6121=AXIS2_PLACEMENT_3D ( 'NONE', #17048, #7227, #1262 ) ;
#6122=ADVANCED_FACE ( 'NONE', ( #19435 ), #11257, .T. ) ;
#6123=CARTESIAN_POINT ( 'NONE',  ( 1.937849085826861328, 0.000000000000000000, 0.000000000000000000 ) ) ;
#6132=DIRECTION ( 'NONE',  ( -0.000000000000000000, 0.000000000000000000, -1.000000000000000000 ) ) ;
#6135=LINE ( 'NONE', #10741, #1042 ) ;
#6143=CYLINDRICAL_SURFACE ( 'NONE', #7548, 10.00000000000000000 ) ;
#6144=ORIENTED_EDGE ( 'NONE', *, *, #10117, .F. ) ;
#6145=CARTESIAN_POINT ( 'NONE',  ( -10.43924542913431175, 0.000000000000000000, 1.000000000000000000 ) ) ;
#6146=CIRCLE ( 'NONE', #2753, 10.00000000000000000 ) ;
#6147=VERTEX_POINT ( 'NONE', #9490 ) ;
#6153=DIRECTION ( 'NONE',  ( 1.000000000000000000, 0.000000000000000000, 0.000000000000000000 ) ) ;
#6158=CARTESIAN_POINT ( 'NONE',  ( -20.00349085826861995, 0.000000000000000000, 1.000000000000000000 ) ) ;
#6172=CARTESIAN_POINT ( 'NONE',  ( 9.000000000000000000, -9.999999999999991118, 1.000000000000000000 ) ) ;
#6177=DIRECTION ( 'NONE',  ( -1.000000000000000000, 0.000000000000000000, 0.000000000000000000 ) ) ;
#6188=ORIENTED_EDGE ( 'NONE', *, *, #1772, .T. ) ;
#6199=CARTESIAN_POINT ( 'NONE',  ( 8.876396343307449754, 10.00000000000000000, 1.000000000000000000 ) ) ;
#6206=VERTEX_POINT ( 'NONE', #13033 ) ;
#6208=LINE ( 'NONE', #9244, #8716 ) ;
#6211=ORIENTED_EDGE ( 'NONE', *, *, #7357, .T. ) ;
#6216=EDGE_CURVE ( 'NONE', #14649, #17557, #9797, .T. ) ;
#6223=CARTESIAN_POINT ( 'NONE',  ( -15.87779268661489773, 11.64110105645932691, 0.000000000000000000 ) ) ;
#6224=CARTESIAN_POINT ( 'NONE',  ( -11.75209451496117197, 16.00000000000000000, 1.000000000000000000 ) ) ;
#6228=ADVANCED_FACE ( 'NONE', ( #8133 ), #16078, .T. ) ;
#6238=CARTESIAN_POINT ( 'NONE',  ( 0.000000000000000000, 11.64110105645932691, 10.00000000000000000 ) ) ;
#6243=VERTEX_POINT ( 'NONE', #4779 ) ;
#6247=FACE_OUTER_BOUND ( 'NONE', #4344, .T. ) ;
#6250=DIRECTION ( 'NONE',  ( 0.000000000000000000, -1.000000000000000000, 0.000000000000000000 ) ) ;
#6252=FACE_OUTER_BOUND ( 'NONE', #9105, .T. ) ;
#6256=PLANE ( 'NONE',  #17433 ) ;
#6259=CIRCLE ( 'NONE', #17949, 10.00000000000000000 ) ;
#6263=VERTEX_POINT ( 'NONE', #6559 ) ;
#6266=ORIENTED_EDGE ( 'NONE', *, *, #9956, .F. ) ;
#6268=ORIENTED_EDGE ( 'NONE', *, *, #310, .T. ) ;
#6271=DIRECTION ( 'NONE',  ( 0.000000000000000000, 1.000000000000000000, -0.000000000000000000 ) ) ;
#6288=EDGE_CURVE ( 'NONE', #5732, #12390, #6965, .T. ) ;
#6290=VECTOR ( 'NONE', #9089, 1000.000000000000000 ) ;
#6291=ORIENTED_EDGE ( 'NONE', *, *, #7873, .T. ) ;
#6297=CARTESIAN_POINT ( 'NONE',  ( 27.44203811574919882, 0.000000000000000000, 0.000000000000000000 ) ) ;
#6299=LINE ( 'NONE', #6199, #15050 ) ;
#6302=FACE_OUTER_BOUND ( 'NONE', #3777, .T. ) ;
#6304=EDGE_CURVE ( 'NONE', #10907, #6038, #16106, .T. ) ;
#6307=ORIENTED_EDGE ( 'NONE', *, *, #15488, .F. ) ;
#6309=CARTESIAN_POINT ( 'NONE',  ( 10.38119784648305810, -14.00000000000000000, 2.000000000000000000 ) ) ;
#6312=VERTEX_POINT ( 'NONE', #11771 ) ;
#6318=VERTEX_POINT ( 'NONE', #18373 ) ;
#6320=VERTEX_POINT ( 'NONE', #583 ) ;
#6321=DIRECTION ( 'NONE',  ( 1.000000000000000000, 0.000000000000000000, -0.000000000000000000 ) ) ;
#6324=LINE ( 'NONE', #8110, #624 ) ;
#6329=DIRECTION ( 'NONE',  ( 0.000000000000000000, 0.000000000000000000, -1.000000000000000000 ) ) ;
#6332=EDGE_CURVE ( 'NONE', #17187, #11652, #5428, .T. ) ;
#6351=ORIENTED_EDGE ( 'NONE', *, *, #1409, .T. ) ;
#6353=CIRCLE ( 'NONE', #11681, 10.00000000000000000 ) ;
#6360=AXIS2_PLACEMENT_3D ( 'NONE', #12960, #19361, #1882 ) ;
#6362=DIRECTION ( 'NONE',  ( 0.000000000000000000, -0.000000000000000000, 1.000000000000000000 ) ) ;
#6366=DIRECTION ( 'NONE',  ( 1.000000000000000000, 0.000000000000000000, -0.000000000000000000 ) ) ;
#6370=CARTESIAN_POINT ( 'NONE',  ( -0.000000000000000000, 11.64110105645932691, 0.000000000000000000 ) ) ;
#6372=ORIENTED_EDGE ( 'NONE', *, *, #1139, .F. ) ;
#6374=AXIS2_PLACEMENT_3D ( 'NONE', #4464, #2682, #9266 ) ;
#6379=CARTESIAN_POINT ( 'NONE',  ( 0.000000000000000000, 10.00000000000000000, 1.000000000000000000 ) ) ;
#6383=CARTESIAN_POINT ( 'NONE',  ( 3.469446951953523943E-14, 10.00000000000009592, 0.000000000000000000 ) ) ;
#6384=EDGE_LOOP ( 'NONE', ( #11659, #10901, #2450, #8096 ) ) ;
#6390=VECTOR ( 'NONE', #3049, 1000.000000000000000 ) ;
#6393=VECTOR ( 'NONE', #14887, 1000.000000000000000 ) ;
#6401=ORIENTED_EDGE ( 'NONE', *, *, #20235, .F. ) ;
#6405=ORIENTED_EDGE ( 'NONE', *, *, #8813, .T. ) ;
#6406=VECTOR ( 'NONE', #12066, 1000.000000000000000 ) ;
#6408=CARTESIAN_POINT ( 'NONE',  ( 29.18266749954691619, 14.63532295040229059, 0.3390567389149258815 ) ) ;
#6413=FACE_OUTER_BOUND ( 'NONE', #9055, .T. ) ;
#6423=ORIENTED_EDGE ( 'NONE', *, *, #11065, .T. ) ;
#6425=LINE ( 'NONE', #8099, #20087 ) ;
#6431=CYLINDRICAL_SURFACE ( 'NONE', #18707, 10.00000000000000000 ) ;
#6432=ORIENTED_EDGE ( 'NONE', *, *, #8864, .F. ) ;
#6434=CARTESIAN_POINT ( 'NONE',  ( -1.734723475976795735E-14, 10.00000000000004619, 1.000000000000000000 ) ) ;
#6436=ADVANCED_FACE ( 'NONE', ( #20353 ), #13950, .T. ) ;
#6441=CARTESIAN_POINT ( 'NONE',  ( 0.000000000000000000, 11.64110105645932691, 10.00000000000000000 ) ) ;
#6444=EDGE_CURVE ( 'NONE', #13250, #14757, #17612, .T. ) ;
#6455=ORIENTED_EDGE ( 'NONE', *, *, #227, .T. ) ;
#6458=ORIENTED_EDGE ( 'NONE', *, *, #10516, .T. ) ;
#6459=ORIENTED_EDGE ( 'NONE', *, *, #9109, .F. ) ;
#6464=ADVANCED_FACE ( 'NONE', ( #9463 ), #14160, .F. ) ;
#6466=EDGE_CURVE ( 'NONE', #16994, #10660, #16050, .T. ) ;
#6470=DIRECTION ( 'NONE',  ( 0.000000000000000000, 1.000000000000000000, 0.000000000000000000 ) ) ;
#6479=CARTESIAN_POINT ( 'NONE',  ( -30.00000000000000000, 3.000000000000000000, 1.000000000000000000 ) ) ;
#6484=ORIENTED_EDGE ( 'NONE', *, *, #330, .T. ) ;
#6500=EDGE_CURVE ( 'NONE', #10101, #2830, #246, .T. ) ;
#6501=DIRECTION ( 'NONE',  ( 1.156482317317871133E-15, 1.000000000000000000, 0.000000000000000000 ) ) ;
#6506=VERTEX_POINT ( 'NONE', #1612 ) ;
#6509=CARTESIAN_POINT ( 'NONE',  ( -0.000000000000000000, 10.00000000000000000, 0.000000000000000000 ) ) ;
#6514=CARTESIAN_POINT ( 'NONE',  ( -15.00000000000000000, 3.000000000000000000, 2.000000000000000000 ) ) ;
#6517=CARTESIAN_POINT ( 'NONE',  ( -7.626396343307448866, 0.000000000000000000, 1.000000000000000000 ) ) ;
#6518=DIRECTION ( 'NONE',  ( 1.000000000000000000, 1.156482317317871971E-16, 0.000000000000000000 ) ) ;
#6526=CARTESIAN_POINT ( 'NONE',  ( 30.80549002841696904, 5.431839045955454637, 0.000000000000000000 ) ) ;
#6535=ORIENTED_EDGE ( 'NONE', *, *, #5016, .F. ) ;
#6537=DIRECTION ( 'NONE',  ( -0.000000000000000000, -0.000000000000000000, -1.000000000000000000 ) ) ;
#6542=LINE ( 'NONE', #6642, #11846 ) ;
#6543=CARTESIAN_POINT ( 'NONE',  ( -27.00000000000000000, 3.000000000000000000, 1.000000000000000000 ) ) ;
#6545=LINE ( 'NONE', #15845, #7650 ) ;
#6550=ADVANCED_FACE ( 'NONE', ( #17826 ), #1512, .F. ) ;
#6555=VERTEX_POINT ( 'NONE', #19097 ) ;
#6557=DIRECTION ( 'NONE',  ( 1.000000000000000000, 0.000000000000000000, 0.000000000000000000 ) ) ;
#6559=CARTESIAN_POINT ( 'NONE',  ( 10.49999999999999645, -9.999999999999991118, 1.000000000000000000 ) ) ;
#6578=CARTESIAN_POINT ( 'NONE',  ( 0.000000000000000000, 11.64110105645932691, 10.00000000000000000 ) ) ;
#6582=ORIENTED_EDGE ( 'NONE', *, *, #17294, .F. ) ;
#6583=DIRECTION ( 'NONE',  ( 0.000000000000000000, 0.000000000000000000, -1.000000000000000000 ) ) ;
#6588=CARTESIAN_POINT ( 'NONE',  ( 18.44064177244175440, 0.000000000000000000, 0.000000000000000000 ) ) ;
#6589=DIRECTION ( 'NONE',  ( -0.000000000000000000, -0.000000000000000000, -1.000000000000000000 ) ) ;
#6596=EDGE_CURVE ( 'NONE', #12186, #3742, #8108, .T. ) ;
#6602=ORIENTED_EDGE ( 'NONE', *, *, #18102, .F. ) ;
#6603=ORIENTED_EDGE ( 'NONE', *, *, #5995, .T. ) ;
#6605=LINE ( 'NONE', #6509, #14431 ) ;
#6606=FILL_AREA_STYLE_COLOUR ( '', #1675 ) ;
#6611=ADVANCED_FACE ( 'NONE', ( #14364 ), #50, .T. ) ;
#6612=DIRECTION ( 'NONE',  ( 0.000000000000000000, 1.000000000000000000, -0.000000000000000000 ) ) ;
#6615=CARTESIAN_POINT ( 'NONE',  ( 6.813547257480585095, 11.64110105645932691, 10.00000000000000000 ) ) ;
#6619=LINE ( 'NONE', #16441, #6735 ) ;
#6621=CIRCLE ( 'NONE', #7293, 10.00000000000000000 ) ;
#6623=ORIENTED_EDGE ( 'NONE', *, *, #16997, .F. ) ;
#6634=ORIENTED_EDGE ( 'NONE', *, *, #4800, .T. ) ;
#6642=CARTESIAN_POINT ( 'NONE',  ( 10.93924542913430820, 0.000000000000000000, 1.000000000000000000 ) ) ;
#6650=VECTOR ( 'NONE', #2060, 1000.000000000000000 ) ;
#6654=VECTOR ( 'NONE', #2139, 1000.000000000000000 ) ;
#6655=ORIENTED_EDGE ( 'NONE', *, *, #7735, .F. ) ;
#6657=VERTEX_POINT ( 'NONE', #13415 ) ;
#6665=VERTEX_POINT ( 'NONE', #19606 ) ;
#6668=EDGE_CURVE ( 'NONE', #13489, #14060, #16456, .T. ) ;
#6673=EDGE_CURVE ( 'NONE', #12837, #19679, #3590, .T. ) ;
#6683=CARTESIAN_POINT ( 'NONE',  ( 15.06494360078803041, 10.00000000000000000, 0.000000000000000000 ) ) ;
#6695=LINE ( 'NONE', #13065, #20178 ) ;
#6704=PLANE ( 'NONE',  #20437 ) ;
#6706=EDGE_CURVE ( 'NONE', #18372, #6318, #5163, .T. ) ;
#6714=ORIENTED_EDGE ( 'NONE', *, *, #1172, .F. ) ;
#6715=EDGE_LOOP ( 'NONE', ( #11744, #4665, #6742, #5589 ) ) ;
#6717=CARTESIAN_POINT ( 'NONE',  ( -30.00000000000000000, 10.00000000000000000, 1.000000000000000000 ) ) ;
#6730=ORIENTED_EDGE ( 'NONE', *, *, #13240, .T. ) ;
#6735=VECTOR ( 'NONE', #19807, 1000.000000000000000 ) ;
#6741=CARTESIAN_POINT ( 'NONE',  ( -0.1250000000000001110, 11.64110105645932691, 10.00000000000000000 ) ) ;
#6742=ORIENTED_EDGE ( 'NONE', *, *, #17190, .T. ) ;
#6745=FACE_OUTER_BOUND ( 'NONE', #20459, .T. ) ;
#6749=DIRECTION ( 'NONE',  ( -0.000000000000000000, 0.000000000000000000, -1.000000000000000000 ) ) ;
#6762=ORIENTED_EDGE ( 'NONE', *, *, #2620, .F. ) ;
#6768=CARTESIAN_POINT ( 'NONE',  ( -1.437849085826860884, 0.000000000000000000, 1.000000000000000000 ) ) ;
#6775=CARTESIAN_POINT ( 'NONE',  ( 0.000000000000000000, 16.00000000000000000, 1.000000000000000000 ) ) ;
#6777=VECTOR ( 'NONE', #20541, 1000.000000000000000 ) ;
#6787=DIRECTION ( 'NONE',  ( 0.000000000000000000, 1.000000000000000000, 0.000000000000000000 ) ) ;
#6792=CIRCLE ( 'NONE', #20161, 10.00000000000000000 ) ;
#6794=VERTEX_POINT ( 'NONE', #16353 ) ;
#6795=CARTESIAN_POINT ( 'NONE',  ( 23.31633994409548549, 11.64110105645932691, 10.00000000000000000 ) ) ;
#6799=DIRECTION ( 'NONE',  ( -0.000000000000000000, -0.000000000000000000, -1.000000000000000000 ) ) ;
#6815=EDGE_CURVE ( 'NONE', #6038, #10907, #17791, .T. ) ;
#6818=DIRECTION ( 'NONE',  ( 0.000000000000000000, 1.000000000000000000, -0.000000000000000000 ) ) ;
#6825=FACE_OUTER_BOUND ( 'NONE', #18265, .T. ) ;
#6832=ORIENTED_EDGE ( 'NONE', *, *, #1609, .T. ) ;
#6836=ORIENTED_EDGE ( 'NONE', *, *, #8253, .T. ) ;
#6842=DIRECTION ( 'NONE',  ( 0.000000000000000000, -0.000000000000000000, 1.000000000000000000 ) ) ;
#6856=EDGE_CURVE ( 'NONE', #8532, #14522, #9027, .T. ) ;
#6858=VECTOR ( 'NONE', #20666, 1000.000000000000000 ) ;
#6862=LINE ( 'NONE', #19843, #9420 ) ;
#6869=FACE_OUTER_BOUND ( 'NONE', #7693, .T. ) ;
#6875=DIRECTION ( 'NONE',  ( 0.000000000000000000, 0.000000000000000000, -1.000000000000000000 ) ) ;
#6882=LINE ( 'NONE', #11792, #1280 ) ;
#6883=FACE_OUTER_BOUND ( 'NONE', #12490, .T. ) ;
#6885=VECTOR ( 'NONE', #11482, 1000.000000000000000 ) ;
#6887=ORIENTED_EDGE ( 'NONE', *, *, #5137, .T. ) ;
#6890=DIRECTION ( 'NONE',  ( -1.000000000000000000, 0.000000000000000000, 0.000000000000000000 ) ) ;
#6891=EDGE_CURVE ( 'NONE', #4104, #12575, #13614, .T. ) ;
#6893=LINE ( 'NONE', #513, #11142 ) ;
#6897=AXIS2_PLACEMENT_3D ( 'NONE', #14475, #17828, #7995 ) ;
#6901=DIRECTION ( 'NONE',  ( 1.000000000000000000, 0.000000000000000000, -0.000000000000000000 ) ) ;
#6902=FACE_OUTER_BOUND ( 'NONE', #13845, .T. ) ;
#6905=EDGE_LOOP ( 'NONE', ( #17854, #1967, #2880, #17072 ) ) ;
#6906=ORIENTED_EDGE ( 'NONE', *, *, #184, .F. ) ;
#6909=CARTESIAN_POINT ( 'NONE',  ( 0.000000000000000000, 10.00000000000000000, 1.000000000000000000 ) ) ;
#6912=CARTESIAN_POINT ( 'NONE',  ( -4.250698171653726654, 10.00000000000000000, 1.000000000000000000 ) ) ;
#6913=CARTESIAN_POINT ( 'NONE',  ( -0.000000000000000000, 10.00000000000000000, 0.000000000000000000 ) ) ;
#6915=CARTESIAN_POINT ( 'NONE',  ( 0.000000000000000000, 10.00000000000000000, 1.000000000000000000 ) ) ;
#6927=AXIS2_PLACEMENT_3D ( 'NONE', #9749, #6612, #19071 ) ;
#6938=DIRECTION ( 'NONE',  ( 0.000000000000000000, 1.000000000000000000, -0.000000000000000000 ) ) ;
#6939=CARTESIAN_POINT ( 'NONE',  ( 6.063547257480584207, 0.000000000000000000, 1.000000000000000000 ) ) ;
#6941=DIRECTION ( 'NONE',  ( 0.000000000000000000, 0.000000000000000000, -1.000000000000000000 ) ) ;
#6944=AXIS2_PLACEMENT_3D ( 'NONE', #5215, #15147, #6890 ) ;
#6952=ORIENTED_EDGE ( 'NONE', *, *, #3802, .F. ) ;
#6958=CARTESIAN_POINT ( 'NONE',  ( -22.06633994409548194, 10.00000000000000000, 0.000000000000000000 ) ) ;
#6964=VERTEX_POINT ( 'NONE', #20225 ) ;
#6965=LINE ( 'NONE', #10105, #10102 ) ;
#6967=VECTOR ( 'NONE', #9287, 1000.000000000000000 ) ;
#6971=EDGE_CURVE ( 'NONE', #11489, #5953, #20020, .T. ) ;
#6973=PLANE ( 'NONE',  #15324 ) ;
#6976=DIRECTION ( 'NONE',  ( 0.000000000000000000, 1.000000000000000000, 0.000000000000000000 ) ) ;
#6980=CIRCLE ( 'NONE', #19353, 10.00000000000000000 ) ;
#6989=DIRECTION ( 'NONE',  ( 1.000000000000000000, 0.000000000000000000, -0.000000000000000000 ) ) ;
#7003=DIRECTION ( 'NONE',  ( -0.000000000000000000, -0.000000000000000000, -1.000000000000000000 ) ) ;
#7011=DIRECTION ( 'NONE',  ( -1.000000000000000000, 0.000000000000000000, 0.000000000000000000 ) ) ;
#7012=CIRCLE ( 'NONE', #13667, 10.00000000000000000 ) ;
#7013=EDGE_CURVE ( 'NONE', #15113, #17093, #2640, .T. ) ;
#7017=EDGE_LOOP ( 'NONE', ( #11175, #9343, #2055, #3543 ) ) ;
#7018=ORIENTED_EDGE ( 'NONE', *, *, #6288, .T. ) ;
#7020=LINE ( 'NONE', #13387, #4440 ) ;
#7022=ORIENTED_EDGE ( 'NONE', *, *, #4835, .T. ) ;
#7026=CARTESIAN_POINT ( 'NONE',  ( 16.37779268661489596, 0.000000000000000000, 0.000000000000000000 ) ) ;
#7040=PRODUCT_DEFINITION_FORMATION_WITH_SPECIFIED_SOURCE ( 'ANY', '', #18864, .NOT_KNOWN. ) ;
#7044=CARTESIAN_POINT ( 'NONE',  ( -1.437849085826860884, 10.00000000000000000, 0.000000000000000000 ) ) ;
#7046=AXIS2_PLACEMENT_3D ( 'NONE', #20557, #1405, #4537 ) ;
#7049=CARTESIAN_POINT ( 'NONE',  ( 26.69203811574920948, 1.543443504701929706E-14, 0.000000000000000000 ) ) ;
#7053=CARTESIAN_POINT ( 'NONE',  ( -12.50209451496117197, 0.000000000000000000, 0.000000000000000000 ) ) ;
#7054=DIRECTION ( 'NONE',  ( 0.000000000000000000, 0.000000000000000000, -1.000000000000000000 ) ) ;
#7060=DIRECTION ( 'NONE',  ( 0.000000000000000000, -1.000000000000000000, 0.000000000000000000 ) ) ;
#7062=VECTOR ( 'NONE', #18009, 1000.000000000000000 ) ;
#7072=ORIENTED_EDGE ( 'NONE', *, *, #7873, .F. ) ;
#7074=EDGE_CURVE ( 'NONE', #19964, #20408, #13823, .T. ) ;
#7076=DIRECTION ( 'NONE',  ( 0.000000000000000000, 0.000000000000000000, 1.000000000000000000 ) ) ;
#7082=CARTESIAN_POINT ( 'NONE',  ( -6.313547257480587760, 0.000000000000000000, 0.000000000000000000 ) ) ;
#7087=LINE ( 'NONE', #19856, #19658 ) ;
#7089=LINE ( 'NONE', #16802, #12212 ) ;
#7100=ORIENTED_EDGE ( 'NONE', *, *, #594, .F. ) ;
#7103=LINE ( 'NONE', #1312, #14125 ) ;
#7105=DIRECTION ( 'NONE',  ( 1.000000000000000000, 0.000000000000000000, -0.000000000000000000 ) ) ;
#7109=PLANE ( 'NONE',  #13321 ) ;
#7113=CARTESIAN_POINT ( 'NONE',  ( 1.937849085826861328, 10.00000000000000000, 1.000000000000000000 ) ) ;
#7117=ORIENTED_EDGE ( 'NONE', *, *, #14786, .F. ) ;
#7119=CARTESIAN_POINT ( 'NONE',  ( 0.6250000000000005551, 0.000000000000000000, 1.000000000000000000 ) ) ;
#7127=VERTEX_POINT ( 'NONE', #8082 ) ;
#7132=CARTESIAN_POINT ( 'NONE',  ( 0.6250000000000005551, 16.00000000000000000, 1.000000000000000000 ) ) ;
#7133=CARTESIAN_POINT ( 'NONE',  ( 0.000000000000000000, 10.00000000000000000, 1.000000000000000000 ) ) ;
#7134=CYLINDRICAL_SURFACE ( 'NONE', #16319, 10.00000000000000000 ) ;
#7138=EDGE_CURVE ( 'NONE', #2445, #2409, #4726, .T. ) ;
#7152=DIRECTION ( 'NONE',  ( 0.000000000000000000, 1.000000000000000000, 0.000000000000000000 ) ) ;
#7156=FACE_OUTER_BOUND ( 'NONE', #8056, .T. ) ;
#7158=CARTESIAN_POINT ( 'NONE',  ( 0.000000000000000000, 10.00000000000000000, 1.000000000000000000 ) ) ;
#7161=CARTESIAN_POINT ( 'NONE',  ( 2.687849085826861995, 10.00000000000000000, 1.000000000000000000 ) ) ;
#7167=ORIENTED_EDGE ( 'NONE', *, *, #11460, .T. ) ;
#7172=ORIENTED_EDGE ( 'NONE', *, *, #7601, .T. ) ;
#7181=FACE_OUTER_BOUND ( 'NONE', #19276, .T. ) ;
#7182=DIRECTION ( 'NONE',  ( -0.000000000000000000, -0.000000000000000000, -1.000000000000000000 ) ) ;
#7184=DIRECTION ( 'NONE',  ( -0.000000000000000000, 0.000000000000000000, 1.000000000000000000 ) ) ;
#7189=DIRECTION ( 'NONE',  ( -1.000000000000000000, 0.000000000000000000, 0.000000000000000000 ) ) ;
#7194=ORIENTED_EDGE ( 'NONE', *, *, #16202, .T. ) ;
#7195=ADVANCED_FACE ( 'NONE', ( #17484 ), #5037, .T. ) ;
#7199=EDGE_CURVE ( 'NONE', #4996, #20631, #2950, .T. ) ;
#7204=AXIS2_PLACEMENT_3D ( 'NONE', #12735, #15564, #3023 ) ;
#7205=ORIENTED_EDGE ( 'NONE', *, *, #15555, .T. ) ;
#7206=DIRECTION ( 'NONE',  ( 1.040834085586084454E-15, 1.000000000000000000, 0.000000000000000000 ) ) ;
#7207=LINE ( 'NONE', #20078, #14278 ) ;
#7210=DIRECTION ( 'NONE',  ( 0.000000000000000000, -1.000000000000000000, 0.000000000000000000 ) ) ;
#7216=VERTEX_POINT ( 'NONE', #11008 ) ;
#7218=LINE ( 'NONE', #1046, #8420 ) ;
#7223=ORIENTED_EDGE ( 'NONE', *, *, #1872, .F. ) ;
#7226=ORIENTED_EDGE ( 'NONE', *, *, #8211, .F. ) ;
#7227=DIRECTION ( 'NONE',  ( 1.000000000000000000, 0.000000000000000000, -0.000000000000000000 ) ) ;
#7228=VECTOR ( 'NONE', #13799, 1000.000000000000000 ) ;
#7232=FACE_OUTER_BOUND ( 'NONE', #19296, .T. ) ;
#7235=EDGE_CURVE ( 'NONE', #18752, #13489, #13233, .T. ) ;
#7236=DIRECTION ( 'NONE',  ( 1.000000000000000000, 0.000000000000000000, 0.000000000000000000 ) ) ;
#7255=DIRECTION ( 'NONE',  ( 0.000000000000000000, 1.000000000000000000, -0.000000000000000000 ) ) ;
#7257=DIRECTION ( 'NONE',  ( 0.000000000000000000, 1.000000000000000000, -0.000000000000000000 ) ) ;
#7262=CARTESIAN_POINT ( 'NONE',  ( 30.00000000000000000, 3.000000000000000000, 1.000000000000000000 ) ) ;
#7273=CARTESIAN_POINT ( 'NONE',  ( -4.250698171653726654, 0.000000000000000000, 1.000000000000000000 ) ) ;
#7274=EDGE_LOOP ( 'NONE', ( #3819, #19124, #2720, #13936 ) ) ;
#7277=DIRECTION ( 'NONE',  ( 0.000000000000000000, -1.000000000000000000, 0.000000000000000000 ) ) ;
#7285=DIRECTION ( 'NONE',  ( 1.000000000000000000, -0.000000000000000000, 0.000000000000000000 ) ) ;
#7287=DIRECTION ( 'NONE',  ( -0.000000000000000000, -0.000000000000000000, -1.000000000000000000 ) ) ;
#7288=CARTESIAN_POINT ( 'NONE',  ( 16.37779268661489596, 11.64110105645932691, 10.00000000000000000 ) ) ;
#7290=DIRECTION ( 'NONE',  ( 0.000000000000000000, 0.000000000000000000, -1.000000000000000000 ) ) ;
#7293=AXIS2_PLACEMENT_3D ( 'NONE', #5506, #10215, #3628 ) ;
#7298=CIRCLE ( 'NONE', #9632, 10.00000000000000000 ) ;
#7299=CARTESIAN_POINT ( 'NONE',  ( -1.437849085826860884, 10.00000000000000000, 1.000000000000000000 ) ) ;
#7300=CARTESIAN_POINT ( 'NONE',  ( 27.94203811574921659, 9.999999999999998224, 1.000000000000000000 ) ) ;
#7301=ORIENTED_EDGE ( 'NONE', *, *, #20162, .T. ) ;
#7302=VERTEX_POINT ( 'NONE', #634 ) ;
#7303=EDGE_CURVE ( 'NONE', #10724, #6116, #3104, .T. ) ;
#7304=ORIENTED_EDGE ( 'NONE', *, *, #9518, .T. ) ;
#7311=CARTESIAN_POINT ( 'NONE',  ( -8.376396343307449754, 16.00000000000000000, 1.000000000000000000 ) ) ;
#7318=ORIENTED_EDGE ( 'NONE', *, *, #5673, .F. ) ;
#7324=CARTESIAN_POINT ( 'NONE',  ( -10.43924542913431175, 11.64110105645932691, 0.000000000000000000 ) ) ;
#7326=VERTEX_POINT ( 'NONE', #8279 ) ;
#7333=LINE ( 'NONE', #18116, #5023 ) ;
#7336=VECTOR ( 'NONE', #14603, 1000.000000000000000 ) ;
#7341=AXIS2_PLACEMENT_3D ( 'NONE', #13715, #16957, #9023 ) ;
#7342=DIRECTION ( 'NONE',  ( 1.000000000000000000, 0.000000000000000000, -0.000000000000000000 ) ) ;
#7353=CARTESIAN_POINT ( 'NONE',  ( 8.876396343307449754, 16.00000000000000000, 1.000000000000000000 ) ) ;
#7356=ORIENTED_EDGE ( 'NONE', *, *, #14763, .T. ) ;
#7357=EDGE_CURVE ( 'NONE', #8920, #11466, #6792, .T. ) ;
#7359=CIRCLE ( 'NONE', #1006, 10.00000000000000000 ) ;
#7362=CARTESIAN_POINT ( 'NONE',  ( 15.00000000000000355, -5.999999999999996447, 1.000000000000000000 ) ) ;
#7367=DIRECTION ( 'NONE',  ( 0.000000000000000000, 1.000000000000000000, 0.000000000000000000 ) ) ;
#7376=AXIS2_PLACEMENT_3D ( 'NONE', #12095, #18486, #12404 ) ;
#7382=VERTEX_POINT ( 'NONE', #7132 ) ;
#7383=ORIENTED_EDGE ( 'NONE', *, *, #14739, .T. ) ;
#7389=CIRCLE ( 'NONE', #14725, 10.00000000000000000 ) ;
#7390=ORIENTED_EDGE ( 'NONE', *, *, #9739, .T. ) ;
#7391=DIRECTION ( 'NONE',  ( 1.000000000000000000, 0.000000000000000000, -0.000000000000000000 ) ) ;
#7392=CARTESIAN_POINT ( 'NONE',  ( 20.50349085826861995, 11.64110105645932691, 0.000000000000000000 ) ) ;
#7395=CARTESIAN_POINT ( 'NONE',  ( -24.87918902992234393, 10.00000000000000000, 1.000000000000000000 ) ) ;
#7397=CARTESIAN_POINT ( 'NONE',  ( -24.12918902992234393, 16.00000000000000000, 1.000000000000000000 ) ) ;
#7400=CARTESIAN_POINT ( 'NONE',  ( -30.00000000000000000, 3.000000000000000000, 1.000000000000000000 ) ) ;
#7407=ORIENTED_EDGE ( 'NONE', *, *, #18376, .T. ) ;
#7410=EDGE_LOOP ( 'NONE', ( #11492, #10050, #6906, #6144 ) ) ;
#7411=AXIS2_PLACEMENT_3D ( 'NONE', #1905, #12990, #8288 ) ;
#7423=CARTESIAN_POINT ( 'NONE',  ( -0.000000000000000000, 11.64110105645932691, 0.000000000000000000 ) ) ;
#7433=CARTESIAN_POINT ( 'NONE',  ( -0.000000000000000000, 11.64110105645932691, 0.000000000000000000 ) ) ;
#7435=ORIENTED_EDGE ( 'NONE', *, *, #7717, .T. ) ;
#7439=AXIS2_PLACEMENT_3D ( 'NONE', #11146, #3097, #8115 ) ;
#7440=CARTESIAN_POINT ( 'NONE',  ( 0.000000000000000000, 10.00000000000000000, 1.000000000000000000 ) ) ;
#7443=LINE ( 'NONE', #6080, #235 ) ;
#7444=DIRECTION ( 'NONE',  ( 0.000000000000000000, 0.000000000000000000, 1.000000000000000000 ) ) ;
#7452=CYLINDRICAL_SURFACE ( 'NONE', #13699, 10.00000000000000000 ) ;
#7460=CARTESIAN_POINT ( 'NONE',  ( 0.000000000000000000, 10.00000000000000000, 1.000000000000000000 ) ) ;
#7461=ORIENTED_EDGE ( 'NONE', *, *, #19077, .F. ) ;
#7471=DIRECTION ( 'NONE',  ( -1.000000000000000000, 0.000000000000000000, 0.000000000000000000 ) ) ;
#7478=CARTESIAN_POINT ( 'NONE',  ( 27.94203811574921303, 11.64110105645932691, 10.00000000000000000 ) ) ;
#7481=ORIENTED_EDGE ( 'NONE', *, *, #7939, .T. ) ;
#7487=EDGE_LOOP ( 'NONE', ( #7914, #16075 ) ) ;
#7489=AXIS2_PLACEMENT_3D ( 'NONE', #5998, #4118, #18554 ) ;
#7490=EDGE_CURVE ( 'NONE', #7216, #12080, #10675, .T. ) ;
#7493=CARTESIAN_POINT ( 'NONE',  ( 10.93924542913430820, 0.000000000000000000, 1.000000000000000000 ) ) ;
#7494=DIRECTION ( 'NONE',  ( 1.000000000000000000, 0.000000000000000000, -0.000000000000000000 ) ) ;
#7498=DIRECTION ( 'NONE',  ( 1.000000000000000000, 0.000000000000000000, 0.000000000000000000 ) ) ;
#7500=LINE ( 'NONE', #20368, #10321 ) ;
#7503=CARTESIAN_POINT ( 'NONE',  ( 4.000698171653723101, 11.64110105645932691, 0.000000000000000000 ) ) ;
#7508=ORIENTED_EDGE ( 'NONE', *, *, #4087, .T. ) ;
#7516=ORIENTED_EDGE ( 'NONE', *, *, #16143, .T. ) ;
#7527=CARTESIAN_POINT ( 'NONE',  ( 4.000698171653723101, 11.64110105645932691, 10.00000000000000000 ) ) ;
#7531=CARTESIAN_POINT ( 'NONE',  ( 27.94203811574921659, 9.999999999999998224, 0.000000000000000000 ) ) ;
#7535=AXIS2_PLACEMENT_3D ( 'NONE', #1000, #7391, #19947 ) ;
#7542=ORIENTED_EDGE ( 'NONE', *, *, #8352, .T. ) ;
#7548=AXIS2_PLACEMENT_3D ( 'NONE', #6238, #11058, #15953 ) ;
#7560=CARTESIAN_POINT ( 'NONE',  ( -5.381197846483055436, -6.000000000000000000, 2.000000000000000000 ) ) ;
#7569=ADVANCED_FACE ( 'NONE', ( #4088 ), #15266, .F. ) ;
#7571=DIRECTION ( 'NONE',  ( -0.000000000000000000, -0.000000000000000000, -1.000000000000000000 ) ) ;
#7576=DIRECTION ( 'NONE',  ( -0.000000000000000000, -0.000000000000000000, -1.000000000000000000 ) ) ;
#7582=ORIENTED_EDGE ( 'NONE', *, *, #17515, .T. ) ;
#7583=ORIENTED_EDGE ( 'NONE', *, *, #16202, .F. ) ;
#7584=CARTESIAN_POINT ( 'NONE',  ( 13.00209451496117374, 10.00000000000000000, 0.000000000000000000 ) ) ;
#7587=ADVANCED_FACE ( 'NONE', ( #18527 ), #7637, .T. ) ;
#7588=CARTESIAN_POINT ( 'NONE',  ( -22.81633994409548549, 16.00000000000000000, 1.000000000000000000 ) ) ;
#7590=FACE_OUTER_BOUND ( 'NONE', #14666, .T. ) ;
#7592=LINE ( 'NONE', #20158, #8331 ) ;
#7594=CARTESIAN_POINT ( 'NONE',  ( 15.06494360078803041, 11.64110105645932691, 0.000000000000000000 ) ) ;
#7596=FACE_OUTER_BOUND ( 'NONE', #19175, .T. ) ;
#7597=DIRECTION ( 'NONE',  ( 1.000000000000000000, -3.469446951953491127E-15, 0.000000000000000000 ) ) ;
#7601=EDGE_CURVE ( 'NONE', #18502, #1851, #13590, .T. ) ;
#7604=ORIENTED_EDGE ( 'NONE', *, *, #4237, .T. ) ;
#7608=VERTEX_POINT ( 'NONE', #9206 ) ;
#7610=EDGE_CURVE ( 'NONE', #2724, #11847, #12027, .T. ) ;
#7616=FACE_OUTER_BOUND ( 'NONE', #16226, .T. ) ;
#7618=CARTESIAN_POINT ( 'NONE',  ( 27.94203811574921303, 11.64110105645932691, 0.000000000000000000 ) ) ;
#7626=CARTESIAN_POINT ( 'NONE',  ( -20.00349085826861995, 11.64110105645932691, 10.00000000000000000 ) ) ;
#7631=VERTEX_POINT ( 'NONE', #14008 ) ;
#7633=VECTOR ( 'NONE', #17022, 1000.000000000000000 ) ;
#7637=PLANE ( 'NONE',  #6121 ) ;
#7644=DIRECTION ( 'NONE',  ( 0.000000000000000000, -1.000000000000000000, 0.000000000000000000 ) ) ;
#7650=VECTOR ( 'NONE', #9675, 1000.000000000000000 ) ;
#7653=AXIS2_PLACEMENT_3D ( 'NONE', #20077, #20389, #16917 ) ;
#7661=DIRECTION ( 'NONE',  ( 1.000000000000000000, 0.000000000000000000, 0.000000000000000000 ) ) ;
#7662=AXIS2_PLACEMENT_3D ( 'NONE', #6441, #12806, #13011 ) ;
#7671=LINE ( 'NONE', #20029, #6406 ) ;
#7685=ORIENTED_EDGE ( 'NONE', *, *, #9276, .F. ) ;
#7687=FACE_OUTER_BOUND ( 'NONE', #12180, .T. ) ;
#7688=AXIS2_PLACEMENT_3D ( 'NONE', #10992, #2, #3242 ) ;
#7692=DIRECTION ( 'NONE',  ( 0.000000000000000000, 1.000000000000000000, -0.000000000000000000 ) ) ;
#7693=EDGE_LOOP ( 'NONE', ( #9298, #7821, #8823, #20097 ) ) ;
#7697=CARTESIAN_POINT ( 'NONE',  ( -0.000000000000000000, 11.64110105645932691, 0.000000000000000000 ) ) ;
#7717=EDGE_CURVE ( 'NONE', #2830, #2924, #11186, .T. ) ;
#7722=VECTOR ( 'NONE', #20212, 1000.000000000000000 ) ;
#7724=CARTESIAN_POINT ( 'NONE',  ( 25.37918902992234393, 0.000000000000000000, 0.000000000000000000 ) ) ;
#7729=LINE ( 'NONE', #6158, #5575 ) ;
#7735=EDGE_CURVE ( 'NONE', #6964, #13772, #1465, .T. ) ;
#7740=VERTEX_POINT ( 'NONE', #4501 ) ;
#7744=ORIENTED_EDGE ( 'NONE', *, *, #10013, .F. ) ;
#7747=CARTESIAN_POINT ( 'NONE',  ( -8.376396343307449754, 0.000000000000000000, 0.000000000000000000 ) ) ;
#7758=EDGE_CURVE ( 'NONE', #4108, #19480, #9511, .T. ) ;
#7767=CARTESIAN_POINT ( 'NONE',  ( -16.62779268661489951, 16.00000000000000000, 1.000000000000000000 ) ) ;
#7771=ORIENTED_EDGE ( 'NONE', *, *, #10492, .F. ) ;
#7785=ORIENTED_EDGE ( 'NONE', *, *, #9483, .T. ) ;
#7787=DIRECTION ( 'NONE',  ( 1.000000000000000000, 0.000000000000000000, -0.000000000000000000 ) ) ;
#7796=ORIENTED_EDGE ( 'NONE', *, *, #18103, .T. ) ;
#7800=PLANE ( 'NONE',  #8972 ) ;
#7801=CARTESIAN_POINT ( 'NONE',  ( -9.689245429134309973, 16.00000000000000000, 1.000000000000000000 ) ) ;
#7802=FACE_OUTER_BOUND ( 'NONE', #12179, .T. ) ;
#7803=FACE_OUTER_BOUND ( 'NONE', #16483, .T. ) ;
#7805=CARTESIAN_POINT ( 'NONE',  ( -24.12918902992234393, 11.64110105645932691, 0.000000000000000000 ) ) ;
#7806=CARTESIAN_POINT ( 'NONE',  ( 10.93924542913430820, 10.00000000000000000, 1.000000000000000000 ) ) ;
#7807=CYLINDRICAL_SURFACE ( 'NONE', #13293, 10.00000000000000000 ) ;
#7808=FACE_OUTER_BOUND ( 'NONE', #12207, .T. ) ;
#7819=ORIENTED_EDGE ( 'NONE', *, *, #5577, .T. ) ;
#7821=ORIENTED_EDGE ( 'NONE', *, *, #18109, .T. ) ;
#7823=FACE_OUTER_BOUND ( 'NONE', #19961, .T. ) ;
#7828=EDGE_CURVE ( 'NONE', #16888, #7956, #16103, .T. ) ;
#7831=CARTESIAN_POINT ( 'NONE',  ( 7.500000000000002665, -9.999999999999991118, 2.000000000000000000 ) ) ;
#7833=ORIENTED_EDGE ( 'NONE', *, *, #1962, .T. ) ;
#7837=VERTEX_POINT ( 'NONE', #20519 ) ;
#7855=CARTESIAN_POINT ( 'NONE',  ( -27.94203811574922725, 3.231447299068595019E-14, 1.000000000000000000 ) ) ;
#7869=EDGE_CURVE ( 'NONE', #6263, #11591, #13793, .T. ) ;
#7870=VECTOR ( 'NONE', #4685, 1000.000000000000000 ) ;
#7872=LINE ( 'NONE', #6297, #13675 ) ;
#7873=EDGE_CURVE ( 'NONE', #12771, #1689, #12540, .T. ) ;
#7877=LINE ( 'NONE', #3071, #12737 ) ;
#7881=ORIENTED_EDGE ( 'NONE', *, *, #13362, .F. ) ;
#7890=DIRECTION ( 'NONE',  ( 0.000000000000000000, 0.000000000000000000, -1.000000000000000000 ) ) ;
#7892=ORIENTED_EDGE ( 'NONE', *, *, #1239, .F. ) ;
#7893=DIRECTION ( 'NONE',  ( -0.000000000000000000, 0.000000000000000000, -1.000000000000000000 ) ) ;
#7894=CARTESIAN_POINT ( 'NONE',  ( -22.81633994409548549, 0.000000000000000000, 1.000000000000000000 ) ) ;
#7895=ORIENTED_EDGE ( 'NONE', *, *, #4493, .F. ) ;
#7898=DIRECTION ( 'NONE',  ( 1.000000000000000000, 0.000000000000000000, 0.000000000000000000 ) ) ;
#7901=DIRECTION ( 'NONE',  ( 0.000000000000000000, -0.000000000000000000, -1.000000000000000000 ) ) ;
#7905=CARTESIAN_POINT ( 'NONE',  ( -4.250698171653726654, 16.00000000000000000, 1.000000000000000000 ) ) ;
#7909=ADVANCED_FACE ( 'NONE', ( #7938, #16303, #10132 ), #11494, .T. ) ;
#7911=VERTEX_POINT ( 'NONE', #5116 ) ;
#7913=PLANE ( 'NONE',  #3678 ) ;
#7914=ORIENTED_EDGE ( 'NONE', *, *, #11381, .T. ) ;
#7915=CARTESIAN_POINT ( 'NONE',  ( -3.500698171653725765, 10.00000000000000000, 1.000000000000000000 ) ) ;
#7924=DIRECTION ( 'NONE',  ( 0.000000000000000000, -1.000000000000000000, 0.000000000000000000 ) ) ;
#7927=ORIENTED_EDGE ( 'NONE', *, *, #3614, .T. ) ;
#7929=DIRECTION ( 'NONE',  ( 0.000000000000000000, 0.000000000000000000, -1.000000000000000000 ) ) ;
#7932=EDGE_CURVE ( 'NONE', #5732, #19679, #20496, .T. ) ;
#7935=VERTEX_POINT ( 'NONE', #14621 ) ;
#7937=ORIENTED_EDGE ( 'NONE', *, *, #17975, .F. ) ;
#7938=FACE_BOUND ( 'NONE', #145, .T. ) ;
#7939=EDGE_CURVE ( 'NONE', #9894, #17687, #1784, .T. ) ;
#7955=STYLED_ITEM ( 'NONE', ( #394 ), #18044 ) ;
#7956=VERTEX_POINT ( 'NONE', #201 ) ;
#7962=ORIENTED_EDGE ( 'NONE', *, *, #6444, .F. ) ;
#7963=CARTESIAN_POINT ( 'NONE',  ( 29.71062960567705602, 11.64110105645932691, 0.000000000000000000 ) ) ;
#7964=DIRECTION ( 'NONE',  ( 0.000000000000000000, 0.000000000000000000, -1.000000000000000000 ) ) ;
#7967=VECTOR ( 'NONE', #18402, 1000.000000000000000 ) ;
#7979=CARTESIAN_POINT ( 'NONE',  ( 27.44203811574919882, 10.00000000000000000, 0.000000000000000000 ) ) ;
#7980=EDGE_CURVE ( 'NONE', #1638, #1689, #3646, .T. ) ;
#7995=DIRECTION ( 'NONE',  ( 0.000000000000000000, 0.000000000000000000, 1.000000000000000000 ) ) ;
#7996=FACE_OUTER_BOUND ( 'NONE', #13103, .T. ) ;
#7998=CARTESIAN_POINT ( 'NONE',  ( 4.000698171653723101, 0.000000000000000000, 1.000000000000000000 ) ) ;
#8002=DIRECTION ( 'NONE',  ( 0.000000000000000000, 1.000000000000000000, 0.000000000000000000 ) ) ;
#8004=AXIS2_PLACEMENT_3D ( 'NONE', #19817, #13820, #4311 ) ;
#8014=ORIENTED_EDGE ( 'NONE', *, *, #6856, .F. ) ;
#8031=AXIS2_PLACEMENT_3D ( 'NONE', #1587, #19178, #3260 ) ;
#8038=DIRECTION ( 'NONE',  ( 1.000000000000000000, 0.000000000000000000, 0.000000000000000000 ) ) ;
#8046=VERTEX_POINT ( 'NONE', #7588 ) ;
#8047=AXIS2_PLACEMENT_3D ( 'NONE', #18367, #3821, #4231 ) ;
#8052=DIRECTION ( 'NONE',  ( -1.000000000000000000, 0.000000000000000000, 0.000000000000000000 ) ) ;
#8056=EDGE_LOOP ( 'NONE', ( #6401, #6458, #18053, #11581 ) ) ;
#8059=CIRCLE ( 'NONE', #13390, 2.999999999999999112 ) ;
#8063=EDGE_CURVE ( 'NONE', #7740, #6147, #2879, .T. ) ;
#8069=CARTESIAN_POINT ( 'NONE',  ( 17.12779268661489596, 11.64110105645932691, 0.000000000000000000 ) ) ;
#8082=CARTESIAN_POINT ( 'NONE',  ( 0.6250000000000005551, 11.64110105645932691, 0.000000000000000000 ) ) ;
#8087=ADVANCED_FACE ( 'NONE', ( #719 ), #12392, .T. ) ;
#8088=DIRECTION ( 'NONE',  ( -1.156482317317871133E-15, -1.000000000000000000, 0.000000000000000000 ) ) ;
#8096=ORIENTED_EDGE ( 'NONE', *, *, #9361, .T. ) ;
#8097=EDGE_CURVE ( 'NONE', #2482, #7326, #7103, .T. ) ;
#8099=CARTESIAN_POINT ( 'NONE',  ( -0.000000000000000000, 10.00000000000000000, 0.000000000000000000 ) ) ;
#8108=LINE ( 'NONE', #17506, #2422 ) ;
#8109=CARTESIAN_POINT ( 'NONE',  ( 0.000000000000000000, 10.00000000000000000, 1.000000000000000000 ) ) ;
#8110=CARTESIAN_POINT ( 'NONE',  ( -13.81494360078803396, 0.000000000000000000, 0.000000000000000000 ) ) ;
#8114=DIRECTION ( 'NONE',  ( -0.000000000000000000, -0.000000000000000000, -1.000000000000000000 ) ) ;
#8115=DIRECTION ( 'NONE',  ( 0.000000000000000000, 0.000000000000000000, -1.000000000000000000 ) ) ;
#8133=FACE_OUTER_BOUND ( 'NONE', #11665, .T. ) ;
#8135=VERTEX_POINT ( 'NONE', #3394 ) ;
#8137=VECTOR ( 'NONE', #18938, 1000.000000000000000 ) ;
#8138=CARTESIAN_POINT ( 'NONE',  ( -29.18266749954690553, 14.63532295040229059, 0.3390567389149233835 ) ) ;
#8144=LINE ( 'NONE', #16088, #14626 ) ;
#8148=VECTOR ( 'NONE', #7277, 1000.000000000000000 ) ;
#8155=CARTESIAN_POINT ( 'NONE',  ( 13.00209451496117374, 0.000000000000000000, 0.000000000000000000 ) ) ;
#8158=ORIENTED_EDGE ( 'NONE', *, *, #118, .T. ) ;
#8163=CARTESIAN_POINT ( 'NONE',  ( -10.49999999999999822, -9.999999999999992895, 2.000000000000000000 ) ) ;
#8171=PLANE ( 'NONE',  #3727 ) ;
#8173=EDGE_CURVE ( 'NONE', #962, #8046, #19201, .T. ) ;
#8180=DIRECTION ( 'NONE',  ( 1.000000000000000000, 0.000000000000000000, 0.000000000000000000 ) ) ;
#8181=VERTEX_POINT ( 'NONE', #4855 ) ;
#8187=PLANE ( 'NONE',  #20050 ) ;
#8189=AXIS2_PLACEMENT_3D ( 'NONE', #14862, #8905, #13396 ) ;
#8195=VERTEX_POINT ( 'NONE', #9667 ) ;
#8205=ORIENTED_EDGE ( 'NONE', *, *, #3529, .T. ) ;
#8211=EDGE_CURVE ( 'NONE', #13178, #17919, #15907, .T. ) ;
#8213=FACE_OUTER_BOUND ( 'NONE', #11409, .T. ) ;
#8217=DIRECTION ( 'NONE',  ( 1.000000000000000000, 0.000000000000000000, 0.000000000000000000 ) ) ;
#8231=EDGE_CURVE ( 'NONE', #17224, #10279, #14574, .T. ) ;
#8232=ORIENTED_EDGE ( 'NONE', *, *, #10118, .T. ) ;
#8242=DIRECTION ( 'NONE',  ( 0.000000000000000000, 0.000000000000000000, -1.000000000000000000 ) ) ;
#8250=PLANE ( 'NONE',  #13281 ) ;
#8253=EDGE_CURVE ( 'NONE', #18307, #12822, #3284, .T. ) ;
#8255=AXIS2_PLACEMENT_3D ( 'NONE', #5920, #9066, #900 ) ;
#8261=CARTESIAN_POINT ( 'NONE',  ( -9.000000000000000000, -9.999999999999992895, 2.000000000000000000 ) ) ;
#8269=CARTESIAN_POINT ( 'NONE',  ( 0.000000000000000000, 16.00000000000000000, 1.000000000000000000 ) ) ;
#8272=EDGE_LOOP ( 'NONE', ( #1384, #4803, #3160, #20126 ) ) ;
#8278=EDGE_LOOP ( 'NONE', ( #15513, #15453, #11355, #4535 ) ) ;
#8279=CARTESIAN_POINT ( 'NONE',  ( 1.937849085826861328, 16.00000000000000000, 1.000000000000000000 ) ) ;
#8283=DIRECTION ( 'NONE',  ( 0.000000000000000000, -1.000000000000000000, 0.000000000000000000 ) ) ;
#8284=EDGE_CURVE ( 'NONE', #13535, #15823, #20663, .T. ) ;
#8288=DIRECTION ( 'NONE',  ( 0.000000000000000000, -0.000000000000000000, 1.000000000000000000 ) ) ;
#8292=ORIENTED_EDGE ( 'NONE', *, *, #11710, .T. ) ;
#8297=ORIENTED_EDGE ( 'NONE', *, *, #15091, .F. ) ;
#8304=VECTOR ( 'NONE', #80, 1000.000000000000000 ) ;
#8307=CARTESIAN_POINT ( 'NONE',  ( 0.6250000000000005551, 10.00000000000000000, 1.000000000000000000 ) ) ;
#8310=CARTESIAN_POINT ( 'NONE',  ( 0.000000000000000000, 10.00000000000000000, 1.000000000000000000 ) ) ;
#8312=ADVANCED_FACE ( 'NONE', ( #6745 ), #51, .T. ) ;
#8317=VECTOR ( 'NONE', #18032, 1000.000000000000000 ) ;
#8328=CARTESIAN_POINT ( 'NONE',  ( 27.44203811574919882, 10.00000000000000000, 1.000000000000000000 ) ) ;
#8329=ORIENTED_EDGE ( 'NONE', *, *, #6971, .F. ) ;
#8331=VECTOR ( 'NONE', #9365, 1000.000000000000000 ) ;
#8334=CARTESIAN_POINT ( 'NONE',  ( -5.381197846483055436, -6.000000000000000000, 2.000000000000000000 ) ) ;
#8335=AXIS2_PLACEMENT_3D ( 'NONE', #17581, #3256, #12974 ) ;
#8337=LINE ( 'NONE', #12831, #7336 ) ;
#8340=EDGE_CURVE ( 'NONE', #2700, #12487, #11338, .T. ) ;
#8352=EDGE_CURVE ( 'NONE', #12771, #20538, #9970, .T. ) ;
#8358=VERTEX_POINT ( 'NONE', #4009 ) ;
#8362=LINE ( 'NONE', #5321, #12640 ) ;
#8363=CARTESIAN_POINT ( 'NONE',  ( -12.50209451496117197, 10.00000000000000000, 0.000000000000000000 ) ) ;
#8366=EDGE_CURVE ( 'NONE', #19354, #10019, #17923, .T. ) ;
#8369=CARTESIAN_POINT ( 'NONE',  ( 0.000000000000000000, 11.64110105645932691, 10.00000000000000000 ) ) ;
#8371=VECTOR ( 'NONE', #18537, 1000.000000000000000 ) ;
#8377=PLANE ( 'NONE',  #5411 ) ;
#8386=ADVANCED_FACE ( 'NONE', ( #7156 ), #13520, .T. ) ;
#8397=EDGE_CURVE ( 'NONE', #20714, #14757, #2560, .T. ) ;
#8398=EDGE_CURVE ( 'NONE', #8135, #5810, #3591, .T. ) ;
#8407=CIRCLE ( 'NONE', #16740, 10.00000000000000000 ) ;
#8414=ORIENTED_EDGE ( 'NONE', *, *, #301, .T. ) ;
#8420=VECTOR ( 'NONE', #4178, 1000.000000000000000 ) ;
#8421=CARTESIAN_POINT ( 'NONE',  ( 0.000000000000000000, 11.64110105645932691, 10.00000000000000000 ) ) ;
#8424=LINE ( 'NONE', #13317, #20105 ) ;
#8430=ORIENTED_EDGE ( 'NONE', *, *, #18365, .T. ) ;
#8438=ORIENTED_EDGE ( 'NONE', *, *, #3114, .T. ) ;
#8441=CARTESIAN_POINT ( 'NONE',  ( -27.94203811574921303, 11.64110105645932691, 0.000000000000000000 ) ) ;
#8442=VERTEX_POINT ( 'NONE', #16553 ) ;
#8444=ORIENTED_EDGE ( 'NONE', *, *, #18887, .T. ) ;
#8449=LINE ( 'NONE', #4044, #1615 ) ;
#8451=LINE ( 'NONE', #11986, #1945 ) ;
#8453=LINE ( 'NONE', #12835, #6885 ) ;
#8460=CARTESIAN_POINT ( 'NONE',  ( -9.689245429134309973, 11.64110105645932691, 0.000000000000000000 ) ) ;
#8462=ORIENTED_EDGE ( 'NONE', *, *, #13307, .F. ) ;
#8470=EDGE_CURVE ( 'NONE', #7956, #19341, #5476, .T. ) ;
#8471=CARTESIAN_POINT ( 'NONE',  ( 0.000000000000000000, 16.00000000000000000, 1.000000000000000000 ) ) ;
#8478=DIRECTION ( 'NONE',  ( 1.000000000000000000, 0.000000000000000000, -0.000000000000000000 ) ) ;
#8479=PLANE ( 'NONE',  #3740 ) ;
#8486=DIRECTION ( 'NONE',  ( 0.000000000000000000, 0.000000000000000000, 1.000000000000000000 ) ) ;
#8487=ORIENTED_EDGE ( 'NONE', *, *, #17457, .T. ) ;
#8490=FACE_OUTER_BOUND ( 'NONE', #9251, .T. ) ;
#8511=EDGE_CURVE ( 'NONE', #1283, #15113, #18239, .T. ) ;
#8514=DIRECTION ( 'NONE',  ( 0.000000000000000000, 0.000000000000000000, 1.000000000000000000 ) ) ;
#8515=DIRECTION ( 'NONE',  ( 0.000000000000000000, 1.000000000000000000, 0.000000000000000000 ) ) ;
#8532=VERTEX_POINT ( 'NONE', #20128 ) ;
#8534=LINE ( 'NONE', #269, #11726 ) ;
#8546=CARTESIAN_POINT ( 'NONE',  ( 15.00000000000000000, 3.673940397442059178E-15, 2.000000000000000000 ) ) ;
#8560=ORIENTED_EDGE ( 'NONE', *, *, #7980, .F. ) ;
#8566=LINE ( 'NONE', #12778, #10018 ) ;
#8570=VECTOR ( 'NONE', #9774, 1000.000000000000000 ) ;
#8575=CARTESIAN_POINT ( 'NONE',  ( -30.00000000000000000, 10.00000000000000000, 1.000000000000000000 ) ) ;
#8576=DIRECTION ( 'NONE',  ( 1.000000000000000000, 0.000000000000000000, 0.000000000000000000 ) ) ;
#8579=EDGE_LOOP ( 'NONE', ( #6634, #17065, #9094, #7435, #18976, #454, #6455, #3433, #5369, #13586, #3516, #18542, #10198, #17354, #20515, #12023, #3308, #14592, #4263, #5785, #15576, #14979, #15758, #19305, #10976, #20508, #10587, #1031, #10960, #2431, #4688, #2247, #8158, #11869, #11359, #13433, #17317, #1559, #17747, #1745, #3310, #15566, #5188, #18724, #10080, #10487, #5884, #9995, #20648, #12632, #16550, #20388, #6351, #17940, #13058, #19768, #1536, #2342, #17320, #18892, #12171, #6405, #1766, #1749, #16478, #7194, #4674, #15621, #11688, #1387, #8232, #16573, #19174, #17479, #20344, #19841, #6188, #2174, #14207, #10253, #6484, #11485, #17268, #12868, #18528, #15319, #18886, #16934, #14782, #767, #10778, #9128, #12920, #16916, #19914, #10568, #12134, #10858, #11301, #3847, #14676, #13657, #11210, #7301, #19740, #18311, #16912, #4943, #14852, #15287, #19301, #3492, #8896, #11430, #10178, #2588, #10544, #9191, #2502, #10982 ) ) ;
#8580=ORIENTED_EDGE ( 'NONE', *, *, #9922, .T. ) ;
#8585=EDGE_LOOP ( 'NONE', ( #4205, #16857, #18515, #16958 ) ) ;
#8588=LINE ( 'NONE', #18425, #10984 ) ;
#8597=ADVANCED_FACE ( 'NONE', ( #130 ), #11311, .F. ) ;
#8600=AXIS2_PLACEMENT_3D ( 'NONE', #15481, #20418, #15269 ) ;
#8607=EDGE_CURVE ( 'NONE', #14781, #5093, #14230, .T. ) ;
#8608=DIRECTION ( 'NONE',  ( 0.000000000000000000, 0.000000000000000000, 1.000000000000000000 ) ) ;
#8609=ORIENTED_EDGE ( 'NONE', *, *, #15120, .F. ) ;
#8619=AXIS2_PLACEMENT_3D ( 'NONE', #6578, #12943, #19346 ) ;
#8622=DIRECTION ( 'NONE',  ( 0.000000000000000000, 0.000000000000000000, -1.000000000000000000 ) ) ;
#8639=ORIENTED_EDGE ( 'NONE', *, *, #18109, .F. ) ;
#8647=VECTOR ( 'NONE', #7571, 1000.000000000000000 ) ;
#8657=VERTEX_POINT ( 'NONE', #2616 ) ;
#8661=VECTOR ( 'NONE', #7898, 1000.000000000000000 ) ;
#8664=ADVANCED_FACE ( 'NONE', ( #10678 ), #17051, .T. ) ;
#8671=LINE ( 'NONE', #16601, #9982 ) ;
#8672=CARTESIAN_POINT ( 'NONE',  ( -0.000000000000000000, 10.00000000000000000, 0.000000000000000000 ) ) ;
#8673=LINE ( 'NONE', #1121, #13084 ) ;
#8679=VECTOR ( 'NONE', #14978, 1000.000000000000000 ) ;
#8681=FACE_OUTER_BOUND ( 'NONE', #127, .T. ) ;
#8682=DIRECTION ( 'NONE',  ( 0.000000000000000000, -1.000000000000000000, 0.000000000000000000 ) ) ;
#8687=VERTEX_POINT ( 'NONE', #17251 ) ;
#8691=ORIENTED_EDGE ( 'NONE', *, *, #10521, .F. ) ;
#8693=CARTESIAN_POINT ( 'NONE',  ( 18.44064177244175440, 10.00000000000000000, 0.000000000000000000 ) ) ;
#8695=EDGE_CURVE ( 'NONE', #5420, #14753, #10476, .T. ) ;
#8697=CARTESIAN_POINT ( 'NONE',  ( -26.94203811574920593, 16.00000000000000000, 1.000000000000000000 ) ) ;
#8699=AXIS2_PLACEMENT_3D ( 'NONE', #129, #13088, #11419 ) ;
#8703=PLANE ( 'NONE',  #13067 ) ;
#8710=ORIENTED_EDGE ( 'NONE', *, *, #5137, .F. ) ;
#8713=PLANE ( 'NONE',  #7341 ) ;
#8714=VECTOR ( 'NONE', #15730, 1000.000000000000000 ) ;
#8716=VECTOR ( 'NONE', #1297, 1000.000000000000000 ) ;
#8720=CIRCLE ( 'NONE', #11388, 10.00000000000000000 ) ;
#8723=LINE ( 'NONE', #15093, #9984 ) ;
#8725=LINE ( 'NONE', #773, #12328 ) ;
#8727=CARTESIAN_POINT ( 'NONE',  ( 12.25209451496117197, 11.64110105645932691, 10.00000000000000000 ) ) ;
#8732=CARTESIAN_POINT ( 'NONE',  ( 6.813547257480585095, 10.00000000000000000, 0.000000000000000000 ) ) ;
#8741=ORIENTED_EDGE ( 'NONE', *, *, #1948, .F. ) ;
#8750=EDGE_CURVE ( 'NONE', #18680, #932, #7443, .T. ) ;
#8753=LINE ( 'NONE', #18267, #15674 ) ;
#8761=EDGE_CURVE ( 'NONE', #20538, #10727, #13591, .T. ) ;
#8763=VECTOR ( 'NONE', #3493, 1000.000000000000000 ) ;
#8769=LINE ( 'NONE', #13661, #12957 ) ;
#8777=VECTOR ( 'NONE', #4315, 1000.000000000000000 ) ;
#8787=EDGE_CURVE ( 'NONE', #13083, #13385, #14529, .T. ) ;
#8791=CARTESIAN_POINT ( 'NONE',  ( 0.000000000000000000, 10.00000000000000000, 1.000000000000000000 ) ) ;
#8793=VECTOR ( 'NONE', #4400, 1000.000000000000000 ) ;
#8796=VERTEX_POINT ( 'NONE', #8163 ) ;
#8801=EDGE_LOOP ( 'NONE', ( #18257, #17548, #18733, #4569 ) ) ;
#8808=LINE ( 'NONE', #12037, #43 ) ;
#8813=EDGE_CURVE ( 'NONE', #20051, #8358, #15994, .T. ) ;
#8818=VECTOR ( 'NONE', #2776, 1000.000000000000000 ) ;
#8823=ORIENTED_EDGE ( 'NONE', *, *, #1409, .F. ) ;
#8824=UNCERTAINTY_MEASURE_WITH_UNIT (LENGTH_MEASURE( 1.000000000000000082E-05 ), #16287, 'distance_accuracy_value', 'NONE');
#8825=ORIENTED_EDGE ( 'NONE', *, *, #17975, .T. ) ;
#8830=LINE ( 'NONE', #18552, #2363 ) ;
#8833=DIRECTION ( 'NONE',  ( 0.000000000000000000, 1.000000000000000000, 0.000000000000000000 ) ) ;
#8834=DIRECTION ( 'NONE',  ( 0.000000000000000000, 1.000000000000000000, -0.000000000000000000 ) ) ;
#8843=VERTEX_POINT ( 'NONE', #9514 ) ;
#8851=EDGE_CURVE ( 'NONE', #5957, #15361, #16107, .T. ) ;
#8852=ORIENTED_EDGE ( 'NONE', *, *, #6500, .F. ) ;
#8854=DIRECTION ( 'NONE',  ( 0.000000000000000000, 0.000000000000000000, -1.000000000000000000 ) ) ;
#8857=PLANE ( 'NONE',  #8255 ) ;
#8864=EDGE_CURVE ( 'NONE', #3392, #20119, #19255, .T. ) ;
#8873=ORIENTED_EDGE ( 'NONE', *, *, #5909, .T. ) ;
#8874=VECTOR ( 'NONE', #3738, 1000.000000000000000 ) ;
#8875=ORIENTED_EDGE ( 'NONE', *, *, #13780, .F. ) ;
#8881=DIRECTION ( 'NONE',  ( 1.000000000000000000, 0.000000000000000000, 0.000000000000000000 ) ) ;
#8892=VECTOR ( 'NONE', #15333, 1000.000000000000000 ) ;
#8895=ORIENTED_EDGE ( 'NONE', *, *, #16297, .T. ) ;
#8896=ORIENTED_EDGE ( 'NONE', *, *, #1907, .F. ) ;
#8905=DIRECTION ( 'NONE',  ( 1.000000000000000000, 0.000000000000000000, -0.000000000000000000 ) ) ;
#8907=CARTESIAN_POINT ( 'NONE',  ( -0.000000000000000000, 11.64110105645932691, 0.000000000000000000 ) ) ;
#8909=DIRECTION ( 'NONE',  ( -1.156482317317871331E-15, 1.000000000000000000, -0.000000000000000000 ) ) ;
#8916=ORIENTED_EDGE ( 'NONE', *, *, #19803, .T. ) ;
#8920=VERTEX_POINT ( 'NONE', #9925 ) ;
#8928=FACE_OUTER_BOUND ( 'NONE', #15368, .T. ) ;
#8933=ORIENTED_EDGE ( 'NONE', *, *, #15625, .F. ) ;
#8935=DIRECTION ( 'NONE',  ( -0.000000000000000000, 0.000000000000000000, -1.000000000000000000 ) ) ;
#8943=CARTESIAN_POINT ( 'NONE',  ( -13.81494360078803396, 10.00000000000000000, 0.000000000000000000 ) ) ;
#8944=VERTEX_POINT ( 'NONE', #8363 ) ;
#8948=DIRECTION ( 'NONE',  ( 1.000000000000000000, -0.000000000000000000, 0.000000000000000000 ) ) ;
#8969=EDGE_LOOP ( 'NONE', ( #798, #1976, #17500, #1795 ) ) ;
#8972=AXIS2_PLACEMENT_3D ( 'NONE', #4551, #14367, #52 ) ;
#8973=VERTEX_POINT ( 'NONE', #19873 ) ;
#8974=DIRECTION ( 'NONE',  ( 0.000000000000000000, 0.000000000000000000, 1.000000000000000000 ) ) ;
#8983=EDGE_CURVE ( 'NONE', #1283, #4081, #16820, .T. ) ;
#8984=EDGE_CURVE ( 'NONE', #8181, #16994, #7207, .T. ) ;
#9000=AXIS2_PLACEMENT_3D ( 'NONE', #16892, #20256, #15529 ) ;
#9001=CARTESIAN_POINT ( 'NONE',  ( 5.381197846483058989, -6.000000000000000000, 2.000000000000000000 ) ) ;
#9004=VERTEX_POINT ( 'NONE', #13781 ) ;
#9017=CARTESIAN_POINT ( 'NONE',  ( 6.063547257480584207, 16.00000000000000000, 1.000000000000000000 ) ) ;
#9023=DIRECTION ( 'NONE',  ( 0.000000000000000000, 0.000000000000000000, 1.000000000000000000 ) ) ;
#9024=ORIENTED_EDGE ( 'NONE', *, *, #13835, .F. ) ;
#9027=LINE ( 'NONE', #7560, #18472 ) ;
#9031=ADVANCED_FACE ( 'NONE', ( #10548 ), #20283, .T. ) ;
#9034=CARTESIAN_POINT ( 'NONE',  ( 14.99999999999999645, 3.000000000000003553, 2.000000000000000000 ) ) ;
#9037=DIRECTION ( 'NONE',  ( -1.000000000000000000, 0.000000000000000000, 0.000000000000000000 ) ) ;
#9045=EDGE_CURVE ( 'NONE', #5093, #4793, #2808, .T. ) ;
#9052=ORIENTED_EDGE ( 'NONE', *, *, #16608, .F. ) ;
#9053=ORIENTED_EDGE ( 'NONE', *, *, #8607, .T. ) ;
#9055=EDGE_LOOP ( 'NONE', ( #3803, #9306, #9793, #3091 ) ) ;
#9060=PLANE ( 'NONE',  #13285 ) ;
#9064=LINE ( 'NONE', #7697, #2305 ) ;
#9066=DIRECTION ( 'NONE',  ( 0.000000000000000000, 1.000000000000000000, 0.000000000000000000 ) ) ;
#9073=EDGE_CURVE ( 'NONE', #20665, #2900, #823, .T. ) ;
#9080=LINE ( 'NONE', #16592, #273 ) ;
#9084=ORIENTED_EDGE ( 'NONE', *, *, #11779, .T. ) ;
#9085=PLANE ( 'NONE',  #11000 ) ;
#9089=DIRECTION ( 'NONE',  ( 1.000000000000000000, 0.000000000000000000, 0.000000000000000000 ) ) ;
#9090=DIRECTION ( 'NONE',  ( 0.000000000000000000, -1.000000000000000000, 0.000000000000000000 ) ) ;
#9094=ORIENTED_EDGE ( 'NONE', *, *, #1472, .T. ) ;
#9096=CYLINDRICAL_SURFACE ( 'NONE', #2070, 10.00000000000000000 ) ;
#9100=DIRECTION ( 'NONE',  ( 0.000000000000000000, 1.000000000000000000, -0.000000000000000000 ) ) ;
#9105=EDGE_LOOP ( 'NONE', ( #9380, #6730, #16938, #3258, #19510, #8414, #8444, #19699, #7796, #8205 ) ) ;
#9107=DIRECTION ( 'NONE',  ( -0.000000000000000000, -0.000000000000000000, -1.000000000000000000 ) ) ;
#9109=EDGE_CURVE ( 'NONE', #4154, #12358, #15246, .T. ) ;
#9113=PLANE ( 'NONE',  #15822 ) ;
#9115=DIRECTION ( 'NONE',  ( 0.000000000000000000, 0.000000000000000000, 1.000000000000000000 ) ) ;
#9119=VECTOR ( 'NONE', #13304, 1000.000000000000000 ) ;
#9120=DIRECTION ( 'NONE',  ( 0.000000000000000000, 0.000000000000000000, -1.000000000000000000 ) ) ;
#9122=EDGE_CURVE ( 'NONE', #5545, #1638, #13567, .T. ) ;
#9125=ORIENTED_EDGE ( 'NONE', *, *, #5592, .F. ) ;
#9128=ORIENTED_EDGE ( 'NONE', *, *, #10521, .T. ) ;
#9131=VECTOR ( 'NONE', #13903, 1000.000000000000000 ) ;
#9133=LINE ( 'NONE', #7362, #13305 ) ;
#9135=EDGE_CURVE ( 'NONE', #14087, #4081, #1140, .T. ) ;
#9136=CARTESIAN_POINT ( 'NONE',  ( -6.313547257480587760, 11.64110105645932691, 10.00000000000000000 ) ) ;
#9138=DIRECTION ( 'NONE',  ( 0.000000000000000000, -0.000000000000000000, 1.000000000000000000 ) ) ;
#9140=PLANE ( 'NONE',  #17316 ) ;
#9149=ORIENTED_EDGE ( 'NONE', *, *, #15120, .T. ) ;
#9150=EDGE_CURVE ( 'NONE', #1608, #4154, #18710, .T. ) ;
#9155=LINE ( 'NONE', #10930, #797 ) ;
#9159=ORIENTED_EDGE ( 'NONE', *, *, #310, .F. ) ;
#9162=DIRECTION ( 'NONE',  ( 0.000000000000000000, 0.000000000000000000, 1.000000000000000000 ) ) ;
#9165=DIRECTION ( 'NONE',  ( -1.000000000000000000, 0.000000000000000000, 0.000000000000000000 ) ) ;
#9166=LINE ( 'NONE', #12503, #18328 ) ;
#9176=ORIENTED_EDGE ( 'NONE', *, *, #18360, .F. ) ;
#9191=ORIENTED_EDGE ( 'NONE', *, *, #14872, .F. ) ;
#9206=CARTESIAN_POINT ( 'NONE',  ( 17.12779268661489596, 10.00000000000000000, 1.000000000000000000 ) ) ;
#9207=ORIENTED_EDGE ( 'NONE', *, *, #15684, .T. ) ;
#9208=LINE ( 'NONE', #1062, #15316 ) ;
#9217=LINE ( 'NONE', #15182, #8371 ) ;
#9225=ORIENTED_EDGE ( 'NONE', *, *, #8253, .F. ) ;
#9228=VECTOR ( 'NONE', #9464, 1000.000000000000000 ) ;
#9242=ADVANCED_FACE ( 'NONE', ( #7823 ), #20594, .T. ) ;
#9244=CARTESIAN_POINT ( 'NONE',  ( 8.126396343307449754, 10.00000000000000000, 1.000000000000000000 ) ) ;
#9251=EDGE_LOOP ( 'NONE', ( #10002, #17868, #18883, #17171 ) ) ;
#9253=ORIENTED_EDGE ( 'NONE', *, *, #784, .T. ) ;
#9257=ORIENTED_EDGE ( 'NONE', *, *, #6815, .F. ) ;
#9266=DIRECTION ( 'NONE',  ( 0.000000000000000000, -0.000000000000000000, 1.000000000000000000 ) ) ;
#9272=ORIENTED_EDGE ( 'NONE', *, *, #8397, .T. ) ;
#9276=EDGE_CURVE ( 'NONE', #6794, #12837, #14186, .T. ) ;
#9277=CARTESIAN_POINT ( 'NONE',  ( -20.75349085826862350, 10.00000000000000000, 1.000000000000000000 ) ) ;
#9280=ORIENTED_EDGE ( 'NONE', *, *, #13629, .F. ) ;
#9284=EDGE_CURVE ( 'NONE', #14996, #6964, #11892, .T. ) ;
#9286=CARTESIAN_POINT ( 'NONE',  ( 8.876396343307449754, 0.000000000000000000, 1.000000000000000000 ) ) ;
#9287=DIRECTION ( 'NONE',  ( 0.000000000000000000, -1.000000000000000000, 0.000000000000000000 ) ) ;
#9291=FACE_OUTER_BOUND ( 'NONE', #2493, .T. ) ;
#9294=ORIENTED_EDGE ( 'NONE', *, *, #9045, .F. ) ;
#9298=ORIENTED_EDGE ( 'NONE', *, *, #2983, .T. ) ;
#9306=ORIENTED_EDGE ( 'NONE', *, *, #1609, .F. ) ;
#9309=AXIS2_PLACEMENT_3D ( 'NONE', #14914, #6976, #5196 ) ;
#9314=DIRECTION ( 'NONE',  ( -0.000000000000000000, 0.000000000000000000, -1.000000000000000000 ) ) ;
#9322=EDGE_CURVE ( 'NONE', #10774, #12491, #18917, .T. ) ;
#9328=EDGE_CURVE ( 'NONE', #14057, #12443, #11071, .T. ) ;
#9331=AXIS2_PLACEMENT_3D ( 'NONE', #15296, #14038, #18765 ) ;
#9343=ORIENTED_EDGE ( 'NONE', *, *, #18783, .T. ) ;
#9349=ORIENTED_EDGE ( 'NONE', *, *, #9284, .T. ) ;
#9352=ORIENTED_EDGE ( 'NONE', *, *, #2961, .T. ) ;
#9353=PLANE ( 'NONE',  #15779 ) ;
#9359=EDGE_CURVE ( 'NONE', #10724, #2654, #9392, .T. ) ;
#9361=EDGE_CURVE ( 'NONE', #14781, #7837, #9588, .T. ) ;
#9362=VERTEX_POINT ( 'NONE', #10865 ) ;
#9365=DIRECTION ( 'NONE',  ( 1.000000000000000000, 0.000000000000000000, 0.000000000000000000 ) ) ;
#9380=ORIENTED_EDGE ( 'NONE', *, *, #2204, .T. ) ;
#9381=LINE ( 'NONE', #14180, #11955 ) ;
#9384=ORIENTED_EDGE ( 'NONE', *, *, #18821, .F. ) ;
#9392=LINE ( 'NONE', #17230, #10665 ) ;
#9397=CARTESIAN_POINT ( 'NONE',  ( 22.56633994409548194, 11.64110105645932691, 0.000000000000000000 ) ) ;
#9402=VERTEX_POINT ( 'NONE', #3621 ) ;
#9408=EDGE_CURVE ( 'NONE', #12390, #13746, #15012, .T. ) ;
#9420=VECTOR ( 'NONE', #5710, 1000.000000000000000 ) ;
#9438=VECTOR ( 'NONE', #18211, 1000.000000000000000 ) ;
#9444=LINE ( 'NONE', #4937, #14051 ) ;
#9453=DIRECTION ( 'NONE',  ( 1.000000000000000000, 0.000000000000000000, 0.000000000000000000 ) ) ;
#9459=DIRECTION ( 'NONE',  ( 1.000000000000000000, -0.000000000000000000, 0.000000000000000000 ) ) ;
#9460=EDGE_LOOP ( 'NONE', ( #4880, #14544, #5191, #13361 ) ) ;
#9461=VECTOR ( 'NONE', #9107, 1000.000000000000000 ) ;
#9463=FACE_OUTER_BOUND ( 'NONE', #10362, .T. ) ;
#9464=DIRECTION ( 'NONE',  ( 0.000000000000000000, 1.000000000000000000, -0.000000000000000000 ) ) ;
#9465=ORIENTED_EDGE ( 'NONE', *, *, #14205, .F. ) ;
#9466=VECTOR ( 'NONE', #15476, 1000.000000000000000 ) ;
#9468=DIRECTION ( 'NONE',  ( 0.000000000000000000, 0.000000000000000000, 1.000000000000000000 ) ) ;
#9469=PLANE ( 'NONE',  #19037 ) ;
#9471=CARTESIAN_POINT ( 'NONE',  ( 10.93924542913430820, 16.00000000000000000, 1.000000000000000000 ) ) ;
#9472=LINE ( 'NONE', #11451, #18787 ) ;
#9473=EDGE_CURVE ( 'NONE', #7127, #20463, #17755, .T. ) ;
#9474=CARTESIAN_POINT ( 'NONE',  ( -7.626396343307448866, 10.00000000000000000, 1.000000000000000000 ) ) ;
#9482=ORIENTED_EDGE ( 'NONE', *, *, #5577, .F. ) ;
#9483=EDGE_CURVE ( 'NONE', #8532, #19920, #11366, .T. ) ;
#9485=DIRECTION ( 'NONE',  ( 0.000000000000000000, 0.000000000000000000, 1.000000000000000000 ) ) ;
#9487=ADVANCED_FACE ( 'NONE', ( #6869 ), #587, .T. ) ;
#9490=CARTESIAN_POINT ( 'NONE',  ( -18.69064177244175795, 10.00000000000000000, 0.000000000000000000 ) ) ;
#9498=CARTESIAN_POINT ( 'NONE',  ( -10.38119784648305632, -14.00000000000000000, 2.000000000000000000 ) ) ;
#9501=ORIENTED_EDGE ( 'NONE', *, *, #16619, .F. ) ;
#9511=LINE ( 'NONE', #6383, #14800 ) ;
#9512=EDGE_LOOP ( 'NONE', ( #2351, #16990, #9053, #13665 ) ) ;
#9514=CARTESIAN_POINT ( 'NONE',  ( -26.19203811574920593, 16.00000000000000000, 1.000000000000000000 ) ) ;
#9518=EDGE_CURVE ( 'NONE', #12186, #5929, #298, .T. ) ;
#9523=DIRECTION ( 'NONE',  ( -0.000000000000000000, 0.000000000000000000, 1.000000000000000000 ) ) ;
#9536=DIRECTION ( 'NONE',  ( 1.000000000000000000, 0.000000000000000000, -0.000000000000000000 ) ) ;
#9540=DIRECTION ( 'NONE',  ( 1.000000000000000000, 0.000000000000000000, 0.000000000000000000 ) ) ;
#9551=LINE ( 'NONE', #348, #15049 ) ;
#9556=CARTESIAN_POINT ( 'NONE',  ( -6.313547257480587760, 10.00000000000000000, 1.000000000000000000 ) ) ;
#9557=CARTESIAN_POINT ( 'NONE',  ( -0.000000000000000000, 10.00000000000000000, 0.000000000000000000 ) ) ;
#9559=EDGE_CURVE ( 'NONE', #12080, #8135, #16186, .T. ) ;
#9561=CARTESIAN_POINT ( 'NONE',  ( 9.000000000000000000, -9.999999999999991118, 2.000000000000000000 ) ) ;
#9582=CARTESIAN_POINT ( 'NONE',  ( 12.25209451496117197, 0.000000000000000000, 1.000000000000000000 ) ) ;
#9588=LINE ( 'NONE', #4481, #1305 ) ;
#9602=DIRECTION ( 'NONE',  ( -0.000000000000000000, -0.000000000000000000, -1.000000000000000000 ) ) ;
#9615=AXIS2_PLACEMENT_3D ( 'NONE', #12016, #11910, #13579 ) ;
#9620=FACE_OUTER_BOUND ( 'NONE', #8579, .T. ) ;
#9625=VECTOR ( 'NONE', #5407, 1000.000000000000000 ) ;
#9626=VERTEX_POINT ( 'NONE', #5917 ) ;
#9630=CARTESIAN_POINT ( 'NONE',  ( 30.00000000000000000, 0.000000000000000000, 1.000000000000000000 ) ) ;
#9632=AXIS2_PLACEMENT_3D ( 'NONE', #17532, #74, #3211 ) ;
#9634=VERTEX_POINT ( 'NONE', #7392 ) ;
#9638=VECTOR ( 'NONE', #11748, 1000.000000000000000 ) ;
#9647=AXIS2_PLACEMENT_3D ( 'NONE', #15648, #4568, #1335 ) ;
#9648=EDGE_CURVE ( 'NONE', #12998, #13229, #1001, .T. ) ;
#9652=DIRECTION ( 'NONE',  ( 0.000000000000000000, 1.000000000000000000, 0.000000000000000000 ) ) ;
#9660=CARTESIAN_POINT ( 'NONE',  ( -3.500698171653725765, 0.000000000000000000, 0.000000000000000000 ) ) ;
#9661=ORIENTED_EDGE ( 'NONE', *, *, #11698, .F. ) ;
#9662=EDGE_CURVE ( 'NONE', #4337, #17093, #20384, .T. ) ;
#9665=EDGE_CURVE ( 'NONE', #18399, #9362, #12288, .T. ) ;
#9667=CARTESIAN_POINT ( 'NONE',  ( 19.19064177244175440, 11.64110105645932691, 0.000000000000000000 ) ) ;
#9669=LINE ( 'NONE', #3287, #8661 ) ;
#9672=FACE_OUTER_BOUND ( 'NONE', #2981, .T. ) ;
#9675=DIRECTION ( 'NONE',  ( -0.000000000000000000, -0.000000000000000000, -1.000000000000000000 ) ) ;
#9678=CIRCLE ( 'NONE', #659, 1.499999999999998668 ) ;
#9686=LINE ( 'NONE', #5086, #13716 ) ;
#9687=ORIENTED_EDGE ( 'NONE', *, *, #1313, .T. ) ;
#9693=VECTOR ( 'NONE', #434, 1000.000000000000000 ) ;
#9696=CARTESIAN_POINT ( 'NONE',  ( 26.69203811574920238, 10.00000000000000000, 1.000000000000000000 ) ) ;
#9699=CARTESIAN_POINT ( 'NONE',  ( -0.000000000000000000, 11.64110105645932691, 0.000000000000000000 ) ) ;
#9702=CARTESIAN_POINT ( 'NONE',  ( 8.876396343307449754, 0.000000000000000000, 1.000000000000000000 ) ) ;
#9713=PLANE ( 'NONE',  #18647 ) ;
#9719=DIRECTION ( 'NONE',  ( 1.000000000000000000, 0.000000000000000000, 0.000000000000000000 ) ) ;
#9727=VECTOR ( 'NONE', #2621, 1000.000000000000000 ) ;
#9733=DIRECTION ( 'NONE',  ( 1.000000000000000000, 0.000000000000000000, 0.000000000000000000 ) ) ;
#9737=ORIENTED_EDGE ( 'NONE', *, *, #1060, .F. ) ;
#9739=EDGE_CURVE ( 'NONE', #15705, #6243, #8753, .T. ) ;
#9742=FACE_OUTER_BOUND ( 'NONE', #15033, .T. ) ;
#9748=FACE_OUTER_BOUND ( 'NONE', #12154, .T. ) ;
#9749=CARTESIAN_POINT ( 'NONE',  ( 10.38119784648305810, -14.00000000000000000, 2.000000000000000000 ) ) ;
#9751=FACE_OUTER_BOUND ( 'NONE', #4157, .T. ) ;
#9752=DIRECTION ( 'NONE',  ( 1.000000000000000000, 0.000000000000000000, -0.000000000000000000 ) ) ;
#9755=FACE_OUTER_BOUND ( 'NONE', #13578, .T. ) ;
#9758=ADVANCED_FACE ( 'NONE', ( #18377 ), #16794, .T. ) ;
#9765=ORIENTED_EDGE ( 'NONE', *, *, #8851, .T. ) ;
#9768=PLANE ( 'NONE',  #14339 ) ;
#9769=AXIS2_PLACEMENT_3D ( 'NONE', #17199, #16228, #9841 ) ;
#9770=VERTEX_POINT ( 'NONE', #15221 ) ;
#9774=DIRECTION ( 'NONE',  ( 1.000000000000000000, 0.000000000000000000, 0.000000000000000000 ) ) ;
#9775=ORIENTED_EDGE ( 'NONE', *, *, #9284, .F. ) ;
#9776=DIRECTION ( 'NONE',  ( 0.000000000000000000, -0.000000000000000000, 1.000000000000000000 ) ) ;
#9779=CARTESIAN_POINT ( 'NONE',  ( 10.18924542913430820, 11.64110105645932691, 10.00000000000000000 ) ) ;
#9780=ADVANCED_FACE ( 'NONE', ( #5717 ), #4140, .T. ) ;
#9786=EDGE_LOOP ( 'NONE', ( #532, #9257 ) ) ;
#9789=AXIS2_PLACEMENT_3D ( 'NONE', #5765, #11922, #5866 ) ;
#9791=ORIENTED_EDGE ( 'NONE', *, *, #20680, .F. ) ;
#9793=ORIENTED_EDGE ( 'NONE', *, *, #19128, .T. ) ;
#9796=ORIENTED_EDGE ( 'NONE', *, *, #18506, .F. ) ;
#9797=LINE ( 'NONE', #176, #1747 ) ;
#9804=CARTESIAN_POINT ( 'NONE',  ( -10.43924542913431175, 11.64110105645932691, 10.00000000000000000 ) ) ;
#9806=CARTESIAN_POINT ( 'NONE',  ( -7.626396343307448866, 10.00000000000000000, 1.000000000000000000 ) ) ;
#9811=ORIENTED_EDGE ( 'NONE', *, *, #16297, .F. ) ;
#9815=ORIENTED_EDGE ( 'NONE', *, *, #16308, .F. ) ;
#9829=FACE_OUTER_BOUND ( 'NONE', #18882, .T. ) ;
#9838=VERTEX_POINT ( 'NONE', #20571 ) ;
#9841=DIRECTION ( 'NONE',  ( 0.000000000000000000, 0.000000000000000000, 1.000000000000000000 ) ) ;
#9842=( NAMED_UNIT ( * ) SI_UNIT ( $, .STERADIAN. ) SOLID_ANGLE_UNIT ( ) );
#9844=VERTEX_POINT ( 'NONE', #1317 ) ;
#9854=CARTESIAN_POINT ( 'NONE',  ( 0.000000000000000000, 11.64110105645932691, 10.00000000000000000 ) ) ;
#9857=EDGE_LOOP ( 'NONE', ( #18187, #14305, #9125, #15104 ) ) ;
#9866=PLANE ( 'NONE',  #11668 ) ;
#9867=ORIENTED_EDGE ( 'NONE', *, *, #13582, .T. ) ;
#9871=EDGE_CURVE ( 'NONE', #19457, #2445, #1215, .T. ) ;
#9873=FACE_OUTER_BOUND ( 'NONE', #9857, .T. ) ;
#9875=CARTESIAN_POINT ( 'NONE',  ( -0.000000000000000000, 10.00000000000000000, 0.000000000000000000 ) ) ;
#9877=DIRECTION ( 'NONE',  ( 0.000000000000000000, 0.000000000000000000, 1.000000000000000000 ) ) ;
#9880=CARTESIAN_POINT ( 'NONE',  ( 16.37779268661489596, 11.64110105645932691, 0.000000000000000000 ) ) ;
#9894=VERTEX_POINT ( 'NONE', #6223 ) ;
#9896=ORIENTED_EDGE ( 'NONE', *, *, #10991, .F. ) ;
#9903=DIRECTION ( 'NONE',  ( -1.000000000000000000, 0.000000000000000000, 0.000000000000000000 ) ) ;
#9908=ADVANCED_FACE ( 'NONE', ( #7802 ), #13956, .T. ) ;
#9915=VECTOR ( 'NONE', #7255, 1000.000000000000000 ) ;
#9916=FACE_OUTER_BOUND ( 'NONE', #16701, .T. ) ;
#9922=EDGE_CURVE ( 'NONE', #10513, #11555, #17699, .T. ) ;
#9925=CARTESIAN_POINT ( 'NONE',  ( 14.31494360078803041, 16.00000000000000000, 1.000000000000000000 ) ) ;
#9931=AXIS2_PLACEMENT_3D ( 'NONE', #14108, #8052, #12847 ) ;
#9934=EDGE_CURVE ( 'NONE', #13997, #193, #8566, .T. ) ;
#9937=LINE ( 'NONE', #1992, #11094 ) ;
#9944=SURFACE_STYLE_USAGE ( .BOTH. , #13082 ) ;
#9945=ORIENTED_EDGE ( 'NONE', *, *, #7717, .F. ) ;
#9956=EDGE_CURVE ( 'NONE', #16247, #7956, #6353, .T. ) ;
#9966=DIRECTION ( 'NONE',  ( 0.000000000000000000, 0.000000000000000000, 1.000000000000000000 ) ) ;
#9967=ORIENTED_EDGE ( 'NONE', *, *, #1099, .T. ) ;
#9970=LINE ( 'NONE', #16458, #9915 ) ;
#9982=VECTOR ( 'NONE', #17026, 1000.000000000000000 ) ;
#9984=VECTOR ( 'NONE', #19411, 1000.000000000000000 ) ;
#9990=CIRCLE ( 'NONE', #5332, 1.499999999999998668 ) ;
#9991=VERTEX_POINT ( 'NONE', #3168 ) ;
#9993=CARTESIAN_POINT ( 'NONE',  ( -0.000000000000000000, 11.64110105645932691, 0.000000000000000000 ) ) ;
#9995=ORIENTED_EDGE ( 'NONE', *, *, #6971, .T. ) ;
#9999=ADVANCED_FACE ( 'NONE', ( #9751 ), #8187, .T. ) ;
#10002=ORIENTED_EDGE ( 'NONE', *, *, #8063, .F. ) ;
#10013=EDGE_CURVE ( 'NONE', #17944, #4108, #7872, .T. ) ;
#10018=VECTOR ( 'NONE', #15814, 1000.000000000000000 ) ;
#10019=VERTEX_POINT ( 'NONE', #1703 ) ;
#10021=CARTESIAN_POINT ( 'NONE',  ( -22.06633994409548194, 0.000000000000000000, 0.000000000000000000 ) ) ;
#10025=ORIENTED_EDGE ( 'NONE', *, *, #1907, .T. ) ;
#10026=VECTOR ( 'NONE', #9090, 1000.000000000000000 ) ;
#10028=ORIENTED_EDGE ( 'NONE', *, *, #9922, .F. ) ;
#10029=EDGE_CURVE ( 'NONE', #7911, #10437, #5323, .T. ) ;
#10030=CYLINDRICAL_SURFACE ( 'NONE', #6944, 1.499999999999996891 ) ;
#10032=CARTESIAN_POINT ( 'NONE',  ( -15.87779268661489773, 0.000000000000000000, 0.000000000000000000 ) ) ;
#10041=VECTOR ( 'NONE', #12193, 1000.000000000000000 ) ;
#10042=ADVANCED_FACE ( 'NONE', ( #6413 ), #14935, .T. ) ;
#10043=ADVANCED_FACE ( 'NONE', ( #11117 ), #15913, .T. ) ;
#10050=ORIENTED_EDGE ( 'NONE', *, *, #20641, .T. ) ;
#10053=ORIENTED_EDGE ( 'NONE', *, *, #9739, .F. ) ;
#10080=ORIENTED_EDGE ( 'NONE', *, *, #9648, .T. ) ;
#10089=DIRECTION ( 'NONE',  ( 0.000000000000000000, -1.000000000000000000, 0.000000000000000000 ) ) ;
#10101=VERTEX_POINT ( 'NONE', #15041 ) ;
#10102=VECTOR ( 'NONE', #5189, 1000.000000000000000 ) ;
#10103=DIRECTION ( 'NONE',  ( 1.000000000000000000, 0.000000000000000000, 0.000000000000000000 ) ) ;
#10105=CARTESIAN_POINT ( 'NONE',  ( 0.000000000000000000, 16.00000000000000000, 1.000000000000000000 ) ) ;
#10117=EDGE_CURVE ( 'NONE', #19407, #2924, #13672, .T. ) ;
#10118=EDGE_CURVE ( 'NONE', #16102, #2930, #11802, .T. ) ;
#10120=CARTESIAN_POINT ( 'NONE',  ( 5.381197846483058989, -6.000000000000000000, 2.000000000000000000 ) ) ;
#10127=CARTESIAN_POINT ( 'NONE',  ( 0.000000000000000000, 10.00000000000000000, 1.000000000000000000 ) ) ;
#10131=VECTOR ( 'NONE', #19558, 1000.000000000000000 ) ;
#10132=FACE_BOUND ( 'NONE', #7487, .T. ) ;
#10141=CARTESIAN_POINT ( 'NONE',  ( 17.12779268661489596, 10.00000000000000000, 1.000000000000000000 ) ) ;
#10143=ADVANCED_FACE ( 'NONE', ( #12008 ), #7109, .T. ) ;
#10148=CARTESIAN_POINT ( 'NONE',  ( 25.37918902992234393, 0.000000000000000000, 1.000000000000000000 ) ) ;
#10151=ORIENTED_EDGE ( 'NONE', *, *, #5330, .F. ) ;
#10154=DIRECTION ( 'NONE',  ( 0.000000000000000000, 1.000000000000000000, 0.000000000000000000 ) ) ;
#10163=LINE ( 'NONE', #6915, #17539 ) ;
#10165=CARTESIAN_POINT ( 'NONE',  ( -17.94064177244175795, 10.00000000000000000, 0.000000000000000000 ) ) ;
#10170=DIRECTION ( 'NONE',  ( -1.000000000000000000, 0.000000000000000000, 0.000000000000000000 ) ) ;
#10177=DIRECTION ( 'NONE',  ( 0.000000000000000000, -1.000000000000000000, 0.000000000000000000 ) ) ;
#10178=ORIENTED_EDGE ( 'NONE', *, *, #4000, .F. ) ;
#10185=FACE_OUTER_BOUND ( 'NONE', #10522, .T. ) ;
#10193=VERTEX_POINT ( 'NONE', #18605 ) ;
#10198=ORIENTED_EDGE ( 'NONE', *, *, #18228, .T. ) ;
#10204=ORIENTED_EDGE ( 'NONE', *, *, #9662, .F. ) ;
#10215=DIRECTION ( 'NONE',  ( -1.000000000000000000, 0.000000000000000000, 0.000000000000000000 ) ) ;
#10226=CARTESIAN_POINT ( 'NONE',  ( -5.381197846483055436, -6.000000000000000000, 1.000000000000000000 ) ) ;
#10227=VERTEX_POINT ( 'NONE', #2592 ) ;
#10231=VERTEX_POINT ( 'NONE', #13884 ) ;
#10236=LINE ( 'NONE', #3760, #16149 ) ;
#10238=CARTESIAN_POINT ( 'NONE',  ( -14.56494360078803396, 10.00000000000000000, 0.000000000000000000 ) ) ;
#10244=DIRECTION ( 'NONE',  ( 0.000000000000000000, 0.000000000000000000, 1.000000000000000000 ) ) ;
#10245=EDGE_CURVE ( 'NONE', #4291, #378, #8671, .T. ) ;
#10253=ORIENTED_EDGE ( 'NONE', *, *, #4405, .T. ) ;
#10256=VECTOR ( 'NONE', #16651, 1000.000000000000000 ) ;
#10258=DIRECTION ( 'NONE',  ( 0.000000000000000000, 1.000000000000000000, 0.000000000000000000 ) ) ;
#10276=CIRCLE ( 'NONE', #3585, 9.999999999999998224 ) ;
#10277=FACE_OUTER_BOUND ( 'NONE', #2972, .T. ) ;
#10279=VERTEX_POINT ( 'NONE', #1242 ) ;
#10281=DIRECTION ( 'NONE',  ( 0.000000000000000000, 0.000000000000000000, 1.000000000000000000 ) ) ;
#10284=ADVANCED_FACE ( 'NONE', ( #7616 ), #13984, .T. ) ;
#10297=ADVANCED_FACE ( 'NONE', ( #6247 ), #4785, .T. ) ;
#10308=AXIS2_PLACEMENT_3D ( 'NONE', #805, #7189, #5611 ) ;
#10319=VECTOR ( 'NONE', #4882, 1000.000000000000000 ) ;
#10321=VECTOR ( 'NONE', #16898, 1000.000000000000000 ) ;
#10332=LINE ( 'NONE', #20071, #17966 ) ;
#10334=ORIENTED_EDGE ( 'NONE', *, *, #19626, .T. ) ;
#10335=VECTOR ( 'NONE', #13419, 1000.000000000000000 ) ;
#10338=ORIENTED_EDGE ( 'NONE', *, *, #718, .F. ) ;
#10341=CARTESIAN_POINT ( 'NONE',  ( 6.063547257480584207, 0.000000000000000000, 1.000000000000000000 ) ) ;
#10350=VECTOR ( 'NONE', #2747, 1000.000000000000000 ) ;
#10357=CARTESIAN_POINT ( 'NONE',  ( 5.381197846483058989, -14.00000000000000000, 1.000000000000000000 ) ) ;
#10362=EDGE_LOOP ( 'NONE', ( #16505, #9765, #10539, #12209, #7407 ) ) ;
#10365=LINE ( 'NONE', #6913, #14642 ) ;
#10372=CARTESIAN_POINT ( 'NONE',  ( 10.38119784648305810, -14.00000000000000000, 2.000000000000000000 ) ) ;
#10395=DIRECTION ( 'NONE',  ( 0.4999999999999947820, 0.8660254037844417052, -0.000000000000000000 ) ) ;
#10396=EDGE_CURVE ( 'NONE', #18054, #3979, #19026, .T. ) ;
#10414=ADVANCED_FACE ( 'NONE', ( #5942 ), #18819, .T. ) ;
#10415=ORIENTED_EDGE ( 'NONE', *, *, #8284, .F. ) ;
#10418=EDGE_LOOP ( 'NONE', ( #11442, #12438, #14904, #7205 ) ) ;
#10424=CARTESIAN_POINT ( 'NONE',  ( 0.000000000000000000, 11.64110105645932691, 10.00000000000000000 ) ) ;
#10435=AXIS2_PLACEMENT_3D ( 'NONE', #9561, #6537, #1922 ) ;
#10437=VERTEX_POINT ( 'NONE', #18713 ) ;
#10442=DIRECTION ( 'NONE',  ( 0.4999999999999949485, -0.8660254037844415942, 0.000000000000000000 ) ) ;
#10443=DIRECTION ( 'NONE',  ( 0.000000000000000000, 0.000000000000000000, 1.000000000000000000 ) ) ;
#10449=LINE ( 'NONE', #7724, #14308 ) ;
#10456=LINE ( 'NONE', #13476, #14695 ) ;
#10471=FACE_OUTER_BOUND ( 'NONE', #240, .T. ) ;
#10472=ORIENTED_EDGE ( 'NONE', *, *, #11522, .F. ) ;
#10473=CARTESIAN_POINT ( 'NONE',  ( 4.750698171653723989, 0.000000000000000000, 0.000000000000000000 ) ) ;
#10475=CARTESIAN_POINT ( 'NONE',  ( -6.313547257480587760, 16.00000000000000000, 1.000000000000000000 ) ) ;
#10476=LINE ( 'NONE', #16942, #12924 ) ;
#10479=FACE_OUTER_BOUND ( 'NONE', #20655, .T. ) ;
#10481=DIRECTION ( 'NONE',  ( 1.000000000000000000, 0.000000000000000000, 0.000000000000000000 ) ) ;
#10487=ORIENTED_EDGE ( 'NONE', *, *, #16771, .T. ) ;
#10492=EDGE_CURVE ( 'NONE', #4793, #19224, #2652, .T. ) ;
#10500=DIRECTION ( 'NONE',  ( -0.000000000000000000, -0.000000000000000000, -1.000000000000000000 ) ) ;
#10502=LINE ( 'NONE', #7262, #8647 ) ;
#10512=CARTESIAN_POINT ( 'NONE',  ( -0.000000000000000000, 11.64110105645932691, 0.000000000000000000 ) ) ;
#10513=VERTEX_POINT ( 'NONE', #3527 ) ;
#10516=EDGE_CURVE ( 'NONE', #14721, #7382, #490, .T. ) ;
#10520=EDGE_CURVE ( 'NONE', #17919, #13894, #16190, .T. ) ;
#10521=EDGE_CURVE ( 'NONE', #1742, #3392, #8337, .T. ) ;
#10522=EDGE_LOOP ( 'NONE', ( #13098, #6952, #9967, #16012 ) ) ;
#10527=CARTESIAN_POINT ( 'NONE',  ( 27.44203811574919882, 0.000000000000000000, 1.000000000000000000 ) ) ;
#10530=LINE ( 'NONE', #18798, #10041 ) ;
#10539=ORIENTED_EDGE ( 'NONE', *, *, #2066, .F. ) ;
#10542=DIRECTION ( 'NONE',  ( -0.000000000000000000, 0.000000000000000000, -1.000000000000000000 ) ) ;
#10543=CIRCLE ( 'NONE', #16212, 10.00000000000000000 ) ;
#10544=ORIENTED_EDGE ( 'NONE', *, *, #1338, .F. ) ;
#10548=FACE_OUTER_BOUND ( 'NONE', #4471, .T. ) ;
#10551=CARTESIAN_POINT ( 'NONE',  ( 0.000000000000000000, 16.00000000000000000, 1.000000000000000000 ) ) ;
#10553=DIRECTION ( 'NONE',  ( -0.000000000000000000, -0.000000000000000000, -1.000000000000000000 ) ) ;
#10562=AXIS2_PLACEMENT_3D ( 'NONE', #2068, #285, #6875 ) ;
#10568=ORIENTED_EDGE ( 'NONE', *, *, #10682, .T. ) ;
#10570=DIRECTION ( 'NONE',  ( -0.000000000000000000, -0.000000000000000000, -1.000000000000000000 ) ) ;
#10571=ORIENTED_EDGE ( 'NONE', *, *, #20314, .F. ) ;
#10575=DIRECTION ( 'NONE',  ( -0.000000000000000000, -0.000000000000000000, -1.000000000000000000 ) ) ;
#10587=ORIENTED_EDGE ( 'NONE', *, *, #16308, .T. ) ;
#10589=CARTESIAN_POINT ( 'NONE',  ( 0.6250000000000005551, 10.00000000000000000, 0.000000000000000000 ) ) ;
#10596=DIRECTION ( 'NONE',  ( -1.000000000000000000, 0.000000000000000000, 0.000000000000000000 ) ) ;
#10597=LINE ( 'NONE', #15405, #13208 ) ;
#10606=LINE ( 'NONE', #2969, #16060 ) ;
#10612=CARTESIAN_POINT ( 'NONE',  ( 0.000000000000000000, 16.00000000000000000, 1.000000000000000000 ) ) ;
#10613=ORIENTED_EDGE ( 'NONE', *, *, #8851, .F. ) ;
#10615=CARTESIAN_POINT ( 'NONE',  ( 21.25349085826861995, 0.000000000000000000, 0.000000000000000000 ) ) ;
#10616=ORIENTED_EDGE ( 'NONE', *, *, #3410, .T. ) ;
#10621=CIRCLE ( 'NONE', #4946, 10.00000000000000000 ) ;
#10622=DIRECTION ( 'NONE',  ( 0.000000000000000000, 1.000000000000000000, -0.000000000000000000 ) ) ;
#10634=VECTOR ( 'NONE', #17956, 1000.000000000000000 ) ;
#10639=EDGE_LOOP ( 'NONE', ( #17301, #6603, #2921, #12071 ) ) ;
#10641=AXIS2_PLACEMENT_3D ( 'NONE', #9582, #11060, #10752 ) ;
#10649=CARTESIAN_POINT ( 'NONE',  ( 24.62918902992234038, 10.00000000000000000, 1.000000000000000000 ) ) ;
#10654=AXIS2_PLACEMENT_3D ( 'NONE', #1138, #17228, #8974 ) ;
#10660=VERTEX_POINT ( 'NONE', #14039 ) ;
#10664=VECTOR ( 'NONE', #1518, 1000.000000000000000 ) ;
#10665=VECTOR ( 'NONE', #14502, 1000.000000000000000 ) ;
#10669=ORIENTED_EDGE ( 'NONE', *, *, #13881, .F. ) ;
#10675=LINE ( 'NONE', #10473, #8793 ) ;
#10676=ORIENTED_EDGE ( 'NONE', *, *, #1139, .T. ) ;
#10678=FACE_OUTER_BOUND ( 'NONE', #3604, .T. ) ;
#10680=VECTOR ( 'NONE', #13854, 1000.000000000000000 ) ;
#10682=EDGE_CURVE ( 'NONE', #6243, #19704, #10597, .T. ) ;
#10684=EDGE_CURVE ( 'NONE', #18061, #8657, #1396, .T. ) ;
#10694=ORIENTED_EDGE ( 'NONE', *, *, #13595, .F. ) ;
#10697=CARTESIAN_POINT ( 'NONE',  ( 2.687849085826861995, 0.000000000000000000, 0.000000000000000000 ) ) ;
#10700=ORIENTED_EDGE ( 'NONE', *, *, #3525, .T. ) ;
#10724=VERTEX_POINT ( 'NONE', #14234 ) ;
#10725=EDGE_CURVE ( 'NONE', #3875, #2724, #18868, .T. ) ;
#10726=CARTESIAN_POINT ( 'NONE',  ( 12.25209451496117197, 11.64110105645932691, 0.000000000000000000 ) ) ;
#10727=VERTEX_POINT ( 'NONE', #4529 ) ;
#10734=AXIS2_PLACEMENT_3D ( 'NONE', #15508, #8833, #15407 ) ;
#10741=CARTESIAN_POINT ( 'NONE',  ( -15.00000000000000000, 3.000000000000000000, 2.000000000000000000 ) ) ;
#10747=ORIENTED_EDGE ( 'NONE', *, *, #7610, .T. ) ;
#10749=DIRECTION ( 'NONE',  ( 0.8660254037844415942, 0.4999999999999949485, -0.000000000000000000 ) ) ;
#10750=EDGE_LOOP ( 'NONE', ( #19434, #14397, #501, #2078 ) ) ;
#10751=VECTOR ( 'NONE', #13681, 1000.000000000000000 ) ;
#10752=DIRECTION ( 'NONE',  ( 0.000000000000000000, 0.000000000000000000, 1.000000000000000000 ) ) ;
#10758=CARTESIAN_POINT ( 'NONE',  ( 0.000000000000000000, 11.64110105645932691, 10.00000000000000000 ) ) ;
#10764=AXIS2_PLACEMENT_3D ( 'NONE', #9779, #18998, #14579 ) ;
#10774=VERTEX_POINT ( 'NONE', #17387 ) ;
#10778=ORIENTED_EDGE ( 'NONE', *, *, #13307, .T. ) ;
#10779=ORIENTED_EDGE ( 'NONE', *, *, #6596, .F. ) ;
#10781=DIRECTION ( 'NONE',  ( 1.000000000000000000, 0.000000000000000000, 0.000000000000000000 ) ) ;
#10792=EDGE_CURVE ( 'NONE', #20520, #1608, #12569, .T. ) ;
#10805=ORIENTED_EDGE ( 'NONE', *, *, #9518, .F. ) ;
#10823=ORIENTED_EDGE ( 'NONE', *, *, #9073, .T. ) ;
#10825=LINE ( 'NONE', #13738, #3708 ) ;
#10832=ORIENTED_EDGE ( 'NONE', *, *, #8984, .F. ) ;
#10836=EDGE_CURVE ( 'NONE', #3725, #1633, #14097, .T. ) ;
#10847=EDGE_CURVE ( 'NONE', #14996, #10231, #15771, .T. ) ;
#10849=CARTESIAN_POINT ( 'NONE',  ( 0.000000000000000000, 10.00000000000000000, 1.000000000000000000 ) ) ;
#10850=DIRECTION ( 'NONE',  ( 0.000000000000000000, 0.000000000000000000, 1.000000000000000000 ) ) ;
#10855=VERTEX_POINT ( 'NONE', #1547 ) ;
#10858=ORIENTED_EDGE ( 'NONE', *, *, #20374, .T. ) ;
#10859=DIRECTION ( 'NONE',  ( 0.000000000000000000, -1.000000000000000000, 0.000000000000000000 ) ) ;
#10863=ORIENTED_EDGE ( 'NONE', *, *, #6668, .T. ) ;
#10865=CARTESIAN_POINT ( 'NONE',  ( -30.00000000000000000, 10.00000000000000000, 0.000000000000000000 ) ) ;
#10867=DIRECTION ( 'NONE',  ( 0.000000000000000000, 0.000000000000000000, 1.000000000000000000 ) ) ;
#10868=CARTESIAN_POINT ( 'NONE',  ( -20.00349085826861995, 0.000000000000000000, 0.000000000000000000 ) ) ;
#10869=CARTESIAN_POINT ( 'NONE',  ( -3.500698171653725765, 0.000000000000000000, 1.000000000000000000 ) ) ;
#10871=LINE ( 'NONE', #17340, #1185 ) ;
#10873=EDGE_CURVE ( 'NONE', #5957, #8181, #10871, .T. ) ;
#10878=ORIENTED_EDGE ( 'NONE', *, *, #15279, .T. ) ;
#10883=LINE ( 'NONE', #20203, #13139 ) ;
#10885=VERTEX_POINT ( 'NONE', #17447 ) ;
#10890=CARTESIAN_POINT ( 'NONE',  ( 21.25349085826861995, 10.00000000000000000, 0.000000000000000000 ) ) ;
#10892=LINE ( 'NONE', #3348, #3713 ) ;
#10897=DIRECTION ( 'NONE',  ( 1.000000000000000000, -1.156482317317871133E-15, 0.000000000000000000 ) ) ;
#10901=ORIENTED_EDGE ( 'NONE', *, *, #2957, .T. ) ;
#10902=ADVANCED_FACE ( 'NONE', ( #9291 ), #15666, .T. ) ;
#10904=ADVANCED_FACE ( 'NONE', ( #18924 ), #10969, .T. ) ;
#10907=VERTEX_POINT ( 'NONE', #7831 ) ;
#10912=DIRECTION ( 'NONE',  ( 0.000000000000000000, 0.000000000000000000, 1.000000000000000000 ) ) ;
#10925=ORIENTED_EDGE ( 'NONE', *, *, #15607, .T. ) ;
#10928=ORIENTED_EDGE ( 'NONE', *, *, #4405, .F. ) ;
#10930=CARTESIAN_POINT ( 'NONE',  ( -0.000000000000000000, 10.00000000000000000, 0.000000000000000000 ) ) ;
#10937=PLANE ( 'NONE',  #15673 ) ;
#10941=ADVANCED_FACE ( 'NONE', ( #6252, #14404, #18718 ), #18072, .F. ) ;
#10942=CARTESIAN_POINT ( 'NONE',  ( -30.00000000000000000, 3.000000000000000000, 0.000000000000000000 ) ) ;
#10943=FACE_OUTER_BOUND ( 'NONE', #19523, .T. ) ;
#10955=CARTESIAN_POINT ( 'NONE',  ( 16.37779268661489596, 10.00000000000000000, 0.000000000000000000 ) ) ;
#10956=ORIENTED_EDGE ( 'NONE', *, *, #6030, .F. ) ;
#10960=ORIENTED_EDGE ( 'NONE', *, *, #7138, .T. ) ;
#10969=PLANE ( 'NONE',  #7204 ) ;
#10976=ORIENTED_EDGE ( 'NONE', *, *, #11571, .T. ) ;
#10982=ORIENTED_EDGE ( 'NONE', *, *, #9665, .T. ) ;
#10983=EDGE_CURVE ( 'NONE', #14522, #19324, #396, .T. ) ;
#10984=VECTOR ( 'NONE', #11722, 1000.000000000000000 ) ;
#10991=EDGE_CURVE ( 'NONE', #7631, #16247, #19445, .T. ) ;
#10992=CARTESIAN_POINT ( 'NONE',  ( 8.126396343307449754, 11.64110105645932691, 10.00000000000000000 ) ) ;
#10994=VECTOR ( 'NONE', #5720, 1000.000000000000000 ) ;
#11000=AXIS2_PLACEMENT_3D ( 'NONE', #5843, #1032, #15245 ) ;
#11003=ORIENTED_EDGE ( 'NONE', *, *, #6084, .T. ) ;
#11007=ORIENTED_EDGE ( 'NONE', *, *, #18453, .T. ) ;
#11008=CARTESIAN_POINT ( 'NONE',  ( 4.750698171653723989, 11.64110105645932691, 0.000000000000000000 ) ) ;
#11009=VECTOR ( 'NONE', #14165, 1000.000000000000000 ) ;
#11010=AXIS2_PLACEMENT_3D ( 'NONE', #10424, #2463, #8854 ) ;
#11025=AXIS2_PLACEMENT_3D ( 'NONE', #18094, #19073, #4730 ) ;
#11034=ORIENTED_EDGE ( 'NONE', *, *, #7074, .T. ) ;
#11039=DIRECTION ( 'NONE',  ( 0.000000000000000000, -0.000000000000000000, 1.000000000000000000 ) ) ;
#11041=VERTEX_POINT ( 'NONE', #4888 ) ;
#11042=DIRECTION ( 'NONE',  ( 1.000000000000000000, 0.000000000000000000, 0.000000000000000000 ) ) ;
#11047=DIRECTION ( 'NONE',  ( 1.000000000000000000, 0.000000000000000000, 0.000000000000000000 ) ) ;
#11058=DIRECTION ( 'NONE',  ( 1.000000000000000000, -0.000000000000000000, 0.000000000000000000 ) ) ;
#11060=DIRECTION ( 'NONE',  ( -1.000000000000000000, 0.000000000000000000, 0.000000000000000000 ) ) ;
#11062=CARTESIAN_POINT ( 'NONE',  ( 0.000000000000000000, 10.00000000000000000, 1.000000000000000000 ) ) ;
#11065=EDGE_CURVE ( 'NONE', #12358, #14797, #8453, .T. ) ;
#11066=VECTOR ( 'NONE', #2516, 1000.000000000000000 ) ;
#11067=EDGE_CURVE ( 'NONE', #8973, #15262, #2532, .T. ) ;
#11068=CIRCLE ( 'NONE', #2045, 10.00000000000000000 ) ;
#11071=LINE ( 'NONE', #4576, #16666 ) ;
#11073=DIRECTION ( 'NONE',  ( -1.000000000000000000, 0.000000000000000000, 0.000000000000000000 ) ) ;
#11091=EDGE_CURVE ( 'NONE', #13894, #6206, #11373, .T. ) ;
#11092=ORIENTED_EDGE ( 'NONE', *, *, #18241, .F. ) ;
#11094=VECTOR ( 'NONE', #19573, 1000.000000000000000 ) ;
#11110=PLANE ( 'NONE',  #16684 ) ;
#11113=VERTEX_POINT ( 'NONE', #5201 ) ;
#11114=DIRECTION ( 'NONE',  ( 0.000000000000000000, 0.000000000000000000, -1.000000000000000000 ) ) ;
#11115=CARTESIAN_POINT ( 'NONE',  ( 0.000000000000000000, 10.00000000000000000, 1.000000000000000000 ) ) ;
#11117=FACE_OUTER_BOUND ( 'NONE', #2252, .T. ) ;
#11127=CARTESIAN_POINT ( 'NONE',  ( -10.38119784648305632, -14.00000000000000000, 1.000000000000000000 ) ) ;
#11137=ORIENTED_EDGE ( 'NONE', *, *, #3127, .T. ) ;
#11142=VECTOR ( 'NONE', #5432, 1000.000000000000000 ) ;
#11146=CARTESIAN_POINT ( 'NONE',  ( 0.000000000000000000, 11.64110105645932691, 10.00000000000000000 ) ) ;
#11147=CARTESIAN_POINT ( 'NONE',  ( 0.000000000000000000, 10.00000000000000000, 1.000000000000000000 ) ) ;
#11156=ORIENTED_EDGE ( 'NONE', *, *, #14680, .F. ) ;
#11160=ORIENTED_EDGE ( 'NONE', *, *, #12931, .T. ) ;
#11174=ADVANCED_FACE ( 'NONE', ( #20169 ), #15443, .T. ) ;
#11175=ORIENTED_EDGE ( 'NONE', *, *, #13376, .F. ) ;
#11182=ORIENTED_EDGE ( 'NONE', *, *, #9408, .F. ) ;
#11186=LINE ( 'NONE', #3138, #1445 ) ;
#11191=CARTESIAN_POINT ( 'NONE',  ( 6.813547257480585095, 11.64110105645932691, 0.000000000000000000 ) ) ;
#11193=PLANE ( 'NONE',  #17023 ) ;
#11198=EDGE_CURVE ( 'NONE', #4337, #8442, #2573, .T. ) ;
#11203=VECTOR ( 'NONE', #2759, 1000.000000000000000 ) ;
#11208=DIRECTION ( 'NONE',  ( -0.000000000000000000, 0.000000000000000000, -1.000000000000000000 ) ) ;
#11210=ORIENTED_EDGE ( 'NONE', *, *, #11091, .T. ) ;
#11212=LINE ( 'NONE', #6717, #14712 ) ;
#11213=EDGE_CURVE ( 'NONE', #15304, #8944, #19751, .T. ) ;
#11219=CARTESIAN_POINT ( 'NONE',  ( 8.126396343307449754, 10.00000000000000000, 1.000000000000000000 ) ) ;
#11225=DIRECTION ( 'NONE',  ( 1.000000000000000000, 1.734723475976787570E-15, 0.000000000000000000 ) ) ;
#11238=CARTESIAN_POINT ( 'NONE',  ( -22.81633994409548549, 10.00000000000000000, 1.000000000000000000 ) ) ;
#11252=CARTESIAN_POINT ( 'NONE',  ( 0.000000000000000000, 16.00000000000000000, 1.000000000000000000 ) ) ;
#11255=CARTESIAN_POINT ( 'NONE',  ( 14.99999999999999645, 3.000000000000003553, 2.000000000000000000 ) ) ;
#11257=PLANE ( 'NONE',  #5089 ) ;
#11261=EDGE_CURVE ( 'NONE', #19679, #17944, #7089, .T. ) ;
#11270=ORIENTED_EDGE ( 'NONE', *, *, #11571, .F. ) ;
#11278=ORIENTED_EDGE ( 'NONE', *, *, #18376, .F. ) ;
#11286=ADVANCED_FACE ( 'NONE', ( #13659 ), #6143, .T. ) ;
#11294=CARTESIAN_POINT ( 'NONE',  ( 15.00000000000000355, -5.999999999999996447, 1.000000000000000000 ) ) ;
#11301=ORIENTED_EDGE ( 'NONE', *, *, #13881, .T. ) ;
#11302=EDGE_LOOP ( 'NONE', ( #7604, #18043, #6432, #4085 ) ) ;
#11304=CYLINDRICAL_SURFACE ( 'NONE', #19471, 10.00000000000000000 ) ;
#11305=CARTESIAN_POINT ( 'NONE',  ( -20.75349085826862350, 16.00000000000000000, 1.000000000000000000 ) ) ;
#11311=PLANE ( 'NONE',  #6927 ) ;
#11312=EDGE_CURVE ( 'NONE', #8687, #17482, #1635, .T. ) ;
#11313=ADVANCED_FACE ( 'NONE', ( #20378 ), #2899, .T. ) ;
#11316=VECTOR ( 'NONE', #15301, 1000.000000000000000 ) ;
#11317=CARTESIAN_POINT ( 'NONE',  ( -15.00000000000000000, 3.000000000000000000, 2.000000000000000000 ) ) ;
#11325=DIRECTION ( 'NONE',  ( 1.000000000000000000, 0.000000000000000000, -0.000000000000000000 ) ) ;
#11332=VECTOR ( 'NONE', #3730, 1000.000000000000000 ) ;
#11338=LINE ( 'NONE', #17726, #8570 ) ;
#11347=DIRECTION ( 'NONE',  ( -0.000000000000000000, -0.000000000000000000, -1.000000000000000000 ) ) ;
#11355=ORIENTED_EDGE ( 'NONE', *, *, #13999, .F. ) ;
#11357=DIRECTION ( 'NONE',  ( 0.000000000000000000, 1.000000000000000000, -0.000000000000000000 ) ) ;
#11358=ORIENTED_EDGE ( 'NONE', *, *, #15091, .T. ) ;
#11359=ORIENTED_EDGE ( 'NONE', *, *, #4045, .T. ) ;
#11366=LINE ( 'NONE', #8334, #6650 ) ;
#11370=DIRECTION ( 'NONE',  ( 1.000000000000000000, 0.000000000000000000, 0.000000000000000000 ) ) ;
#11373=LINE ( 'NONE', #16090, #4545 ) ;
#11380=VECTOR ( 'NONE', #3381, 1000.000000000000000 ) ;
#11381=EDGE_CURVE ( 'NONE', #11591, #6263, #14310, .T. ) ;
#11382=CARTESIAN_POINT ( 'NONE',  ( -3.500698171653725765, 11.64110105645932691, 10.00000000000000000 ) ) ;
#11385=ORIENTED_EDGE ( 'NONE', *, *, #330, .F. ) ;
#11386=VECTOR ( 'NONE', #173, 1000.000000000000000 ) ;
#11388=AXIS2_PLACEMENT_3D ( 'NONE', #8727, #13119, #9877 ) ;
#11389=ORIENTED_EDGE ( 'NONE', *, *, #10991, .T. ) ;
#11392=ORIENTED_EDGE ( 'NONE', *, *, #6706, .F. ) ;
#11398=DIRECTION ( 'NONE',  ( 1.000000000000000000, -0.000000000000000000, 0.000000000000000000 ) ) ;
#11404=DIRECTION ( 'NONE',  ( -1.000000000000000000, 0.000000000000000000, 0.000000000000000000 ) ) ;
#11409=EDGE_LOOP ( 'NONE', ( #7461, #15498, #3481, #11564 ) ) ;
#11411=DIRECTION ( 'NONE',  ( 1.000000000000000000, -0.000000000000000000, 0.000000000000000000 ) ) ;
#11412=LINE ( 'NONE', #12872, #9693 ) ;
#11414=VECTOR ( 'NONE', #2820, 1000.000000000000000 ) ;
#11419=DIRECTION ( 'NONE',  ( 0.000000000000000000, 0.000000000000000000, -1.000000000000000000 ) ) ;
#11421=CARTESIAN_POINT ( 'NONE',  ( 0.000000000000000000, 16.00000000000000000, 1.000000000000000000 ) ) ;
#11428=VECTOR ( 'NONE', #16183, 1000.000000000000000 ) ;
#11429=PLANE ( 'NONE',  #2679 ) ;
#11430=ORIENTED_EDGE ( 'NONE', *, *, #16997, .T. ) ;
#11432=DIRECTION ( 'NONE',  ( 0.000000000000000000, 1.000000000000000000, -0.000000000000000000 ) ) ;
#11442=ORIENTED_EDGE ( 'NONE', *, *, #7490, .F. ) ;
#11444=VECTOR ( 'NONE', #4423, 1000.000000000000000 ) ;
#11447=ADVANCED_FACE ( 'NONE', ( #3004 ), #4667, .T. ) ;
#11450=DIRECTION ( 'NONE',  ( -1.000000000000000000, 0.000000000000000000, 0.000000000000000000 ) ) ;
#11451=CARTESIAN_POINT ( 'NONE',  ( -5.381197846483055436, -14.00000000000000000, 1.000000000000000000 ) ) ;
#11459=AXIS2_PLACEMENT_3D ( 'NONE', #13060, #13161, #19352 ) ;
#11460=EDGE_CURVE ( 'NONE', #8046, #12514, #7359, .T. ) ;
#11463=ADVANCED_FACE ( 'NONE', ( #1533 ), #7913, .F. ) ;
#11466=VERTEX_POINT ( 'NONE', #14276 ) ;
#11473=ORIENTED_EDGE ( 'NONE', *, *, #7013, .T. ) ;
#11476=DIRECTION ( 'NONE',  ( -1.000000000000000000, 0.000000000000000000, 0.000000000000000000 ) ) ;
#11482=DIRECTION ( 'NONE',  ( 1.000000000000000000, 0.000000000000000000, 0.000000000000000000 ) ) ;
#11485=ORIENTED_EDGE ( 'NONE', *, *, #9934, .T. ) ;
#11489=VERTEX_POINT ( 'NONE', #11561 ) ;
#11492=ORIENTED_EDGE ( 'NONE', *, *, #15494, .T. ) ;
#11494=PLANE ( 'NONE',  #19836 ) ;
#11495=AXIS2_PLACEMENT_3D ( 'NONE', #876, #15298, #1091 ) ;
#11501=EDGE_CURVE ( 'NONE', #10019, #9838, #1744, .T. ) ;
#11509=FACE_OUTER_BOUND ( 'NONE', #12201, .T. ) ;
#11518=LINE ( 'NONE', #15908, #18065 ) ;
#11522=EDGE_CURVE ( 'NONE', #10727, #9894, #18052, .T. ) ;
#11539=LINE ( 'NONE', #243, #8679 ) ;
#11541=ORIENTED_EDGE ( 'NONE', *, *, #10873, .T. ) ;
#11549=DIRECTION ( 'NONE',  ( 0.000000000000000000, 0.000000000000000000, 1.000000000000000000 ) ) ;
#11555=VERTEX_POINT ( 'NONE', #6958 ) ;
#11561=CARTESIAN_POINT ( 'NONE',  ( -5.563547257480587760, 10.00000000000000000, 0.000000000000000000 ) ) ;
#11563=EDGE_CURVE ( 'NONE', #15857, #17187, #9686, .T. ) ;
#11564=ORIENTED_EDGE ( 'NONE', *, *, #14477, .T. ) ;
#11565=CARTESIAN_POINT ( 'NONE',  ( 0.000000000000000000, 10.00000000000000000, 1.000000000000000000 ) ) ;
#11568=VERTEX_POINT ( 'NONE', #14493 ) ;
#11570=DIRECTION ( 'NONE',  ( 1.000000000000000000, 0.000000000000000000, 0.000000000000000000 ) ) ;
#11571=EDGE_CURVE ( 'NONE', #1689, #10727, #19320, .T. ) ;
#11577=CARTESIAN_POINT ( 'NONE',  ( -22.81633994409548549, 0.000000000000000000, 0.000000000000000000 ) ) ;
#11581=ORIENTED_EDGE ( 'NONE', *, *, #2552, .F. ) ;
#11589=ORIENTED_EDGE ( 'NONE', *, *, #7235, .F. ) ;
#11591=VERTEX_POINT ( 'NONE', #17847 ) ;
#11592=CARTESIAN_POINT ( 'NONE',  ( -0.000000000000000000, 10.00000000000000000, 0.000000000000000000 ) ) ;
#11593=ORIENTED_EDGE ( 'NONE', *, *, #16019, .F. ) ;
#11604=CARTESIAN_POINT ( 'NONE',  ( -0.000000000000000000, 11.64110105645932691, 0.000000000000000000 ) ) ;
#11608=VERTEX_POINT ( 'NONE', #13133 ) ;
#11609=ORIENTED_EDGE ( 'NONE', *, *, #2665, .F. ) ;
#11611=CARTESIAN_POINT ( 'NONE',  ( 4.750698171653723989, 11.64110105645932691, 10.00000000000000000 ) ) ;
#11614=DIRECTION ( 'NONE',  ( -0.000000000000000000, -0.000000000000000000, -1.000000000000000000 ) ) ;
#11615=VECTOR ( 'NONE', #10442, 1000.000000000000000 ) ;
#11618=DIRECTION ( 'NONE',  ( 0.000000000000000000, -1.000000000000000000, 0.000000000000000000 ) ) ;
#11620=CARTESIAN_POINT ( 'NONE',  ( -0.000000000000000000, 10.00000000000000000, 0.000000000000000000 ) ) ;
#11633=DIRECTION ( 'NONE',  ( -0.000000000000000000, 0.000000000000000000, -1.000000000000000000 ) ) ;
#11636=ORIENTED_EDGE ( 'NONE', *, *, #14774, .T. ) ;
#11639=CIRCLE ( 'NONE', #16652, 10.00000000000000000 ) ;
#11643=CARTESIAN_POINT ( 'NONE',  ( -26.19203811574920593, 0.000000000000000000, 0.000000000000000000 ) ) ;
#11644=DIRECTION ( 'NONE',  ( 1.000000000000000000, 0.000000000000000000, 0.000000000000000000 ) ) ;
#11646=LINE ( 'NONE', #8310, #16729 ) ;
#11649=CARTESIAN_POINT ( 'NONE',  ( -5.381197846483055436, -14.00000000000000000, 2.000000000000000000 ) ) ;
#11652=VERTEX_POINT ( 'NONE', #5391 ) ;
#11656=VECTOR ( 'NONE', #3771, 1000.000000000000000 ) ;
#11659=ORIENTED_EDGE ( 'NONE', *, *, #4045, .F. ) ;
#11663=ORIENTED_EDGE ( 'NONE', *, *, #17407, .F. ) ;
#11665=EDGE_LOOP ( 'NONE', ( #10571, #5650, #17400, #676 ) ) ;
#11668=AXIS2_PLACEMENT_3D ( 'NONE', #19603, #16154, #11633 ) ;
#11678=ORIENTED_EDGE ( 'NONE', *, *, #13895, .T. ) ;
#11681=AXIS2_PLACEMENT_3D ( 'NONE', #615, #12879, #2183 ) ;
#11683=DIRECTION ( 'NONE',  ( 1.000000000000000000, 0.000000000000000000, -0.000000000000000000 ) ) ;
#11688=ORIENTED_EDGE ( 'NONE', *, *, #8398, .T. ) ;
#11692=ORIENTED_EDGE ( 'NONE', *, *, #15540, .F. ) ;
#11693=DIRECTION ( 'NONE',  ( 1.000000000000000000, 0.000000000000000000, 0.000000000000000000 ) ) ;
#11698=EDGE_CURVE ( 'NONE', #6312, #17224, #888, .T. ) ;
#11700=CYLINDRICAL_SURFACE ( 'NONE', #18383, 10.00000000000000000 ) ;
#11704=VECTOR ( 'NONE', #11357, 1000.000000000000000 ) ;
#11708=DIRECTION ( 'NONE',  ( 1.000000000000000000, 0.000000000000000000, 0.000000000000000000 ) ) ;
#11710=EDGE_CURVE ( 'NONE', #10231, #10101, #2452, .T. ) ;
#11712=ORIENTED_EDGE ( 'NONE', *, *, #17369, .F. ) ;
#11713=EDGE_CURVE ( 'NONE', #6020, #8442, #19840, .T. ) ;
#11716=DIRECTION ( 'NONE',  ( -1.000000000000000000, 0.000000000000000000, 0.000000000000000000 ) ) ;
#11717=CARTESIAN_POINT ( 'NONE',  ( 22.56633994409548194, 0.000000000000000000, 1.000000000000000000 ) ) ;
#11722=DIRECTION ( 'NONE',  ( 1.000000000000000000, 0.000000000000000000, 0.000000000000000000 ) ) ;
#11726=VECTOR ( 'NONE', #6557, 1000.000000000000000 ) ;
#11729=ADVANCED_FACE ( 'NONE', ( #18157 ), #18259, .T. ) ;
#11730=DIRECTION ( 'NONE',  ( 0.000000000000000000, 0.000000000000000000, -1.000000000000000000 ) ) ;
#11744=ORIENTED_EDGE ( 'NONE', *, *, #11198, .F. ) ;
#11748=DIRECTION ( 'NONE',  ( 0.000000000000000000, 1.000000000000000000, -0.000000000000000000 ) ) ;
#11753=DIRECTION ( 'NONE',  ( 0.000000000000000000, 1.000000000000000000, -0.000000000000000000 ) ) ;
#11766=ORIENTED_EDGE ( 'NONE', *, *, #3855, .T. ) ;
#11767=ORIENTED_EDGE ( 'NONE', *, *, #5453, .T. ) ;
#11768=VECTOR ( 'NONE', #14573, 1000.000000000000000 ) ;
#11771=CARTESIAN_POINT ( 'NONE',  ( -24.87918902992234393, 11.64110105645932691, 0.000000000000000000 ) ) ;
#11779=EDGE_CURVE ( 'NONE', #9991, #346, #18469, .T. ) ;
#11792=CARTESIAN_POINT ( 'NONE',  ( 22.56633994409548194, 0.000000000000000000, 0.000000000000000000 ) ) ;
#11796=ORIENTED_EDGE ( 'NONE', *, *, #1174, .F. ) ;
#11802=LINE ( 'NONE', #2705, #5311 ) ;
#11805=VECTOR ( 'NONE', #8881, 1000.000000000000000 ) ;
#11818=CIRCLE ( 'NONE', #18853, 10.00000000000000000 ) ;
#11830=EDGE_CURVE ( 'NONE', #13, #12186, #15212, .T. ) ;
#11846=VECTOR ( 'NONE', #12903, 1000.000000000000000 ) ;
#11847=VERTEX_POINT ( 'NONE', #9556 ) ;
#11850=DIRECTION ( 'NONE',  ( 0.000000000000000000, 0.000000000000000000, -1.000000000000000000 ) ) ;
#11855=CARTESIAN_POINT ( 'NONE',  ( -26.94203811574920593, 10.00000000000000000, 0.000000000000000000 ) ) ;
#11859=ORIENTED_EDGE ( 'NONE', *, *, #5958, .T. ) ;
#11865=CIRCLE ( 'NONE', #8189, 10.00000000000000000 ) ;
#11869=ORIENTED_EDGE ( 'NONE', *, *, #19487, .T. ) ;
#11879=PLANE ( 'NONE',  #9309 ) ;
#11892=( BOUNDED_CURVE ( )  B_SPLINE_CURVE ( 3, ( #1542, #8138, #17538, #18816 ),
 .UNSPECIFIED., .F., .F. ) 
 B_SPLINE_CURVE_WITH_KNOTS ( ( 4, 4 ),
 ( 1.119769514998634197, 1.570796326794896558 ),
 .UNSPECIFIED. ) 
 CURVE ( )  GEOMETRIC_REPRESENTATION_ITEM ( )  RATIONAL_B_SPLINE_CURVE ( ( 1.000000000000000000, 0.9831196229872642967, 0.9831196229872642967, 1.000000000000000000 ) ) 
 REPRESENTATION_ITEM ( '' )  );
#11894=ORIENTED_EDGE ( 'NONE', *, *, #14069, .F. ) ;
#11899=EDGE_CURVE ( 'NONE', #10437, #6147, #13944, .T. ) ;
#11909=ORIENTED_EDGE ( 'NONE', *, *, #4015, .F. ) ;
#11910=DIRECTION ( 'NONE',  ( -1.000000000000000000, 0.000000000000000000, 0.000000000000000000 ) ) ;
#11915=ORIENTED_EDGE ( 'NONE', *, *, #10029, .F. ) ;
#11922=DIRECTION ( 'NONE',  ( -0.8660254037844417052, 0.4999999999999947264, 0.000000000000000000 ) ) ;
#11947=CARTESIAN_POINT ( 'NONE',  ( 0.000000000000000000, 16.00000000000000000, 1.000000000000000000 ) ) ;
#11950=VECTOR ( 'NONE', #7924, 1000.000000000000000 ) ;
#11951=FACE_OUTER_BOUND ( 'NONE', #2897, .T. ) ;
#11955=VECTOR ( 'NONE', #10859, 1000.000000000000000 ) ;
#11982=AXIS2_PLACEMENT_3D ( 'NONE', #16282, #19329, #276 ) ;
#11985=CIRCLE ( 'NONE', #18363, 10.00000000000000000 ) ;
#11986=CARTESIAN_POINT ( 'NONE',  ( 24.62918902992234038, 0.000000000000000000, 0.000000000000000000 ) ) ;
#11987=VECTOR ( 'NONE', #6153, 1000.000000000000000 ) ;
#11995=ORIENTED_EDGE ( 'NONE', *, *, #3355, .F. ) ;
#12006=CARTESIAN_POINT ( 'NONE',  ( -17.94064177244175795, 0.000000000000000000, 0.000000000000000000 ) ) ;
#12008=FACE_OUTER_BOUND ( 'NONE', #5276, .T. ) ;
#12016=CARTESIAN_POINT ( 'NONE',  ( -6.313547257480587760, 0.000000000000000000, 1.000000000000000000 ) ) ;
#12017=CARTESIAN_POINT ( 'NONE',  ( 0.000000000000000000, 11.64110105645932691, 10.00000000000000000 ) ) ;
#12023=ORIENTED_EDGE ( 'NONE', *, *, #1060, .T. ) ;
#12026=ORIENTED_EDGE ( 'NONE', *, *, #8173, .F. ) ;
#12027=LINE ( 'NONE', #7440, #9131 ) ;
#12034=CARTESIAN_POINT ( 'NONE',  ( -5.563547257480587760, 0.000000000000000000, 1.000000000000000000 ) ) ;
#12037=CARTESIAN_POINT ( 'NONE',  ( 27.94203811574922725, 3.231447299068595019E-14, 1.000000000000000000 ) ) ;
#12054=VERTEX_POINT ( 'NONE', #20167 ) ;
#12059=VECTOR ( 'NONE', #19826, 1000.000000000000000 ) ;
#12061=CARTESIAN_POINT ( 'NONE',  ( -27.00000000000000000, 3.000000000000000000, 0.000000000000000000 ) ) ;
#12065=AXIS2_PLACEMENT_3D ( 'NONE', #7855, #10897, #6501 ) ;
#12066=DIRECTION ( 'NONE',  ( 1.000000000000000000, 0.000000000000000000, 0.000000000000000000 ) ) ;
#12071=ORIENTED_EDGE ( 'NONE', *, *, #8983, .F. ) ;
#12078=CARTESIAN_POINT ( 'NONE',  ( 10.93924542913430820, 10.00000000000000000, 1.000000000000000000 ) ) ;
#12080=VERTEX_POINT ( 'NONE', #5827 ) ;
#12081=CARTESIAN_POINT ( 'NONE',  ( 6.063547257480584207, 10.00000000000000000, 1.000000000000000000 ) ) ;
#12082=VERTEX_POINT ( 'NONE', #903 ) ;
#12087=PLANE ( 'NONE',  #20228 ) ;
#12094=DIRECTION ( 'NONE',  ( 0.000000000000000000, 0.000000000000000000, -1.000000000000000000 ) ) ;
#12095=CARTESIAN_POINT ( 'NONE',  ( 25.37918902992234393, 11.64110105645932691, 10.00000000000000000 ) ) ;
#12097=DIRECTION ( 'NONE',  ( 1.000000000000000000, 0.000000000000000000, 0.000000000000000000 ) ) ;
#12099=CARTESIAN_POINT ( 'NONE',  ( 10.93924542913430820, 0.000000000000000000, 0.000000000000000000 ) ) ;
#12103=ORIENTED_EDGE ( 'NONE', *, *, #15279, .F. ) ;
#12110=VERTEX_POINT ( 'NONE', #7503 ) ;
#12111=ADVANCED_FACE ( 'NONE', ( #12505 ), #15229, .F. ) ;
#12113=DIRECTION ( 'NONE',  ( 0.000000000000000000, 1.000000000000000000, -0.000000000000000000 ) ) ;
#12117=DIRECTION ( 'NONE',  ( 0.000000000000000000, -1.000000000000000000, 0.000000000000000000 ) ) ;
#12119=DIRECTION ( 'NONE',  ( -0.000000000000000000, -0.000000000000000000, -1.000000000000000000 ) ) ;
#12123=ORIENTED_EDGE ( 'NONE', *, *, #6304, .T. ) ;
#12134=ORIENTED_EDGE ( 'NONE', *, *, #1239, .T. ) ;
#12135=EDGE_CURVE ( 'NONE', #10019, #2700, #7012, .T. ) ;
#12140=AXIS2_PLACEMENT_3D ( 'NONE', #8261, #6589, #13165 ) ;
#12153=LINE ( 'NONE', #10697, #13343 ) ;
#12154=EDGE_LOOP ( 'NONE', ( #17429, #17222, #15572, #9661 ) ) ;
#12160=DIRECTION ( 'NONE',  ( -0.000000000000000000, -0.000000000000000000, -1.000000000000000000 ) ) ;
#12163=DIRECTION ( 'NONE',  ( 0.000000000000000000, 0.000000000000000000, 1.000000000000000000 ) ) ;
#12166=EDGE_CURVE ( 'NONE', #8796, #15857, #9678, .T. ) ;
#12171=ORIENTED_EDGE ( 'NONE', *, *, #13999, .T. ) ;
#12179=EDGE_LOOP ( 'NONE', ( #7516, #11160, #11593, #5362 ) ) ;
#12180=EDGE_LOOP ( 'NONE', ( #18701, #18020, #20200, #11909 ) ) ;
#12182=VERTEX_POINT ( 'NONE', #19211 ) ;
#12184=EDGE_CURVE ( 'NONE', #9402, #2930, #14380, .T. ) ;
#12186=VERTEX_POINT ( 'NONE', #7905 ) ;
#12187=CARTESIAN_POINT ( 'NONE',  ( -12.50209451496117197, 10.00000000000000000, 1.000000000000000000 ) ) ;
#12193=DIRECTION ( 'NONE',  ( 0.000000000000000000, -1.000000000000000000, 0.000000000000000000 ) ) ;
#12201=EDGE_LOOP ( 'NONE', ( #3341, #15210, #17753, #6602 ) ) ;
#12205=LINE ( 'NONE', #1023, #11615 ) ;
#12206=CARTESIAN_POINT ( 'NONE',  ( 25.37918902992234393, 10.00000000000000000, 1.000000000000000000 ) ) ;
#12207=EDGE_LOOP ( 'NONE', ( #19528, #17848, #12323, #1357 ) ) ;
#12209=ORIENTED_EDGE ( 'NONE', *, *, #2204, .F. ) ;
#12210=ADVANCED_FACE ( 'NONE', ( #12601 ), #19314, .T. ) ;
#12212=VECTOR ( 'NONE', #19955, 1000.000000000000000 ) ;
#12213=ORIENTED_EDGE ( 'NONE', *, *, #3614, .F. ) ;
#12231=ORIENTED_EDGE ( 'NONE', *, *, #2957, .F. ) ;
#12247=DIRECTION ( 'NONE',  ( 1.000000000000000000, -0.000000000000000000, 0.000000000000000000 ) ) ;
#12253=DIRECTION ( 'NONE',  ( 1.000000000000000000, 0.000000000000000000, 0.000000000000000000 ) ) ;
#12263=FACE_OUTER_BOUND ( 'NONE', #8585, .T. ) ;
#12264=CARTESIAN_POINT ( 'NONE',  ( 24.62918902992234038, 0.000000000000000000, 1.000000000000000000 ) ) ;
#12268=ORIENTED_EDGE ( 'NONE', *, *, #19253, .F. ) ;
#12280=CARTESIAN_POINT ( 'NONE',  ( 8.876396343307449754, 10.00000000000000000, 0.000000000000000000 ) ) ;
#12281=EDGE_LOOP ( 'NONE', ( #20617, #4613, #13557, #7022 ) ) ;
#12283=ADVANCED_FACE ( 'NONE', ( #16637 ), #11429, .T. ) ;
#12284=ADVANCED_FACE ( 'NONE', ( #18226 ), #17814, .T. ) ;
#12286=ORIENTED_EDGE ( 'NONE', *, *, #10245, .F. ) ;
#12287=DIRECTION ( 'NONE',  ( -0.000000000000000000, 0.000000000000000000, -1.000000000000000000 ) ) ;
#12288=LINE ( 'NONE', #2674, #10680 ) ;
#12289=DIRECTION ( 'NONE',  ( 1.000000000000000000, 0.000000000000000000, 0.000000000000000000 ) ) ;
#12293=CARTESIAN_POINT ( 'NONE',  ( 0.000000000000000000, 11.64110105645932691, 10.00000000000000000 ) ) ;
#12311=VECTOR ( 'NONE', #18141, 1000.000000000000000 ) ;
#12312=VERTEX_POINT ( 'NONE', #18329 ) ;
#12313=DIRECTION ( 'NONE',  ( 0.000000000000000000, 0.000000000000000000, -1.000000000000000000 ) ) ;
#12317=CARTESIAN_POINT ( 'NONE',  ( 20.50349085826861995, 16.00000000000000000, 1.000000000000000000 ) ) ;
#12318=CARTESIAN_POINT ( 'NONE',  ( 1.937849085826861328, 10.00000000000000000, 0.000000000000000000 ) ) ;
#12323=ORIENTED_EDGE ( 'NONE', *, *, #5507, .T. ) ;
#12326=DIRECTION ( 'NONE',  ( 0.000000000000000000, -1.000000000000000000, 0.000000000000000000 ) ) ;
#12328=VECTOR ( 'NONE', #5580, 1000.000000000000000 ) ;
#12333=ORIENTED_EDGE ( 'NONE', *, *, #81, .F. ) ;
#12336=LINE ( 'NONE', #18421, #3249 ) ;
#12340=ORIENTED_EDGE ( 'NONE', *, *, #5779, .F. ) ;
#12346=AXIS2_PLACEMENT_3D ( 'NONE', #16646, #5571, #2324 ) ;
#12358=VERTEX_POINT ( 'NONE', #9017 ) ;
#12362=ORIENTED_EDGE ( 'NONE', *, *, #1962, .F. ) ;
#12370=CARTESIAN_POINT ( 'NONE',  ( 0.000000000000000000, 11.64110105645932691, 10.00000000000000000 ) ) ;
#12390=VERTEX_POINT ( 'NONE', #18748 ) ;
#12392=PLANE ( 'NONE',  #3785 ) ;
#12394=DIRECTION ( 'NONE',  ( 1.000000000000000000, 0.000000000000000000, -0.000000000000000000 ) ) ;
#12397=EDGE_CURVE ( 'NONE', #378, #17017, #9217, .T. ) ;
#12399=CARTESIAN_POINT ( 'NONE',  ( 15.06494360078803041, 16.00000000000000000, 1.000000000000000000 ) ) ;
#12403=CARTESIAN_POINT ( 'NONE',  ( -27.00000000000000000, 3.000000000000000000, 1.000000000000000000 ) ) ;
#12404=DIRECTION ( 'NONE',  ( 0.000000000000000000, 0.000000000000000000, -1.000000000000000000 ) ) ;
#12405=DIRECTION ( 'NONE',  ( 1.000000000000000000, 1.156482317317871133E-15, -0.000000000000000000 ) ) ;
#12410=ORIENTED_EDGE ( 'NONE', *, *, #5673, .T. ) ;
#12413=ORIENTED_EDGE ( 'NONE', *, *, #3472, .T. ) ;
#12415=DIRECTION ( 'NONE',  ( -1.000000000000000000, 0.000000000000000000, 0.000000000000000000 ) ) ;
#12416=ORIENTED_EDGE ( 'NONE', *, *, #6815, .T. ) ;
#12425=AXIS2_PLACEMENT_3D ( 'NONE', #160, #3520, #17437 ) ;
#12427=ADVANCED_FACE ( 'NONE', ( #5777 ), #7452, .T. ) ;
#12438=ORIENTED_EDGE ( 'NONE', *, *, #14321, .T. ) ;
#12443=VERTEX_POINT ( 'NONE', #18436 ) ;
#12452=DIRECTION ( 'NONE',  ( -0.000000000000000000, -0.000000000000000000, -1.000000000000000000 ) ) ;
#12487=VERTEX_POINT ( 'NONE', #8069 ) ;
#12490=EDGE_LOOP ( 'NONE', ( #9815, #7481, #3116, #7582 ) ) ;
#12491=VERTEX_POINT ( 'NONE', #11294 ) ;
#12492=LINE ( 'NONE', #6123, #8818 ) ;
#12496=CARTESIAN_POINT ( 'NONE',  ( 0.000000000000000000, 10.00000000000000000, 1.000000000000000000 ) ) ;
#12503=CARTESIAN_POINT ( 'NONE',  ( -15.00000000000000000, 3.000000000000000000, 2.000000000000000000 ) ) ;
#12505=FACE_OUTER_BOUND ( 'NONE', #3110, .T. ) ;
#12514=VERTEX_POINT ( 'NONE', #8 ) ;
#12515=DIRECTION ( 'NONE',  ( 0.000000000000000000, 0.000000000000000000, 1.000000000000000000 ) ) ;
#12516=ORIENTED_EDGE ( 'NONE', *, *, #15509, .F. ) ;
#12520=CARTESIAN_POINT ( 'NONE',  ( -28.94203811574919882, 16.00000000000000000, 1.000000000000000000 ) ) ;
#12525=CARTESIAN_POINT ( 'NONE',  ( 19.19064177244175440, 0.000000000000000000, 0.000000000000000000 ) ) ;
#12529=ORIENTED_EDGE ( 'NONE', *, *, #13519, .F. ) ;
#12540=LINE ( 'NONE', #12749, #8137 ) ;
#12542=EDGE_LOOP ( 'NONE', ( #2099, #11392, #8873, #12410 ) ) ;
#12544=DIRECTION ( 'NONE',  ( 1.000000000000000000, 0.000000000000000000, 0.000000000000000000 ) ) ;
#12567=ADVANCED_FACE ( 'NONE', ( #3152 ), #18851, .T. ) ;
#12569=LINE ( 'NONE', #15816, #4524 ) ;
#12575=VERTEX_POINT ( 'NONE', #19057 ) ;
#12577=LINE ( 'NONE', #19085, #14728 ) ;
#12597=CARTESIAN_POINT ( 'NONE',  ( -17.94064177244175795, 10.00000000000000000, 1.000000000000000000 ) ) ;
#12599=DIRECTION ( 'NONE',  ( 0.000000000000000000, 1.000000000000000000, -0.000000000000000000 ) ) ;
#12601=FACE_OUTER_BOUND ( 'NONE', #17605, .T. ) ;
#12606=ORIENTED_EDGE ( 'NONE', *, *, #17834, .T. ) ;
#12607=EDGE_CURVE ( 'NONE', #16994, #17840, #8059, .T. ) ;
#12610=ORIENTED_EDGE ( 'NONE', *, *, #2928, .F. ) ;
#12630=CARTESIAN_POINT ( 'NONE',  ( -5.381197846483055436, -14.00000000000000000, 2.000000000000000000 ) ) ;
#12632=ORIENTED_EDGE ( 'NONE', *, *, #13629, .T. ) ;
#12636=DIRECTION ( 'NONE',  ( 1.000000000000000000, 0.000000000000000000, 0.000000000000000000 ) ) ;
#12640=VECTOR ( 'NONE', #11693, 1000.000000000000000 ) ;
#12647=CARTESIAN_POINT ( 'NONE',  ( -9.689245429134309973, 0.000000000000000000, 1.000000000000000000 ) ) ;
#12661=ORIENTED_EDGE ( 'NONE', *, *, #14786, .T. ) ;
#12667=AXIS2_PLACEMENT_3D ( 'NONE', #556, #16547, #8608 ) ;
#12670=DIRECTION ( 'NONE',  ( -0.000000000000000000, -0.000000000000000000, -1.000000000000000000 ) ) ;
#12671=ADVANCED_FACE ( 'NONE', ( #9620 ), #6704, .F. ) ;
#12675=DIRECTION ( 'NONE',  ( 0.1736481776669309696, 0.9848077530122080203, 0.000000000000000000 ) ) ;
#12681=EDGE_CURVE ( 'NONE', #8195, #10885, #7389, .T. ) ;
#12683=LINE ( 'NONE', #6526, #3047 ) ;
#12694=ORIENTED_EDGE ( 'NONE', *, *, #8750, .T. ) ;
#12698=CARTESIAN_POINT ( 'NONE',  ( -4.250698171653726654, 10.00000000000000000, 1.000000000000000000 ) ) ;
#12701=DIRECTION ( 'NONE',  ( 0.000000000000000000, 1.000000000000000000, 0.000000000000000000 ) ) ;
#12704=CYLINDRICAL_SURFACE ( 'NONE', #12425, 2.999999999999999112 ) ;
#12706=AXIS2_PLACEMENT_3D ( 'NONE', #14071, #4248, #20479 ) ;
#12717=CARTESIAN_POINT ( 'NONE',  ( 0.000000000000000000, 11.64110105645932691, 10.00000000000000000 ) ) ;
#12720=LINE ( 'NONE', #11565, #19695 ) ;
#12724=VECTOR ( 'NONE', #62, 1000.000000000000000 ) ;
#12730=ADVANCED_FACE ( 'NONE', ( #16518 ), #5024, .T. ) ;
#12735=CARTESIAN_POINT ( 'NONE',  ( 0.000000000000000000, 10.00000000000000000, 1.000000000000000000 ) ) ;
#12737=VECTOR ( 'NONE', #20644, 1000.000000000000000 ) ;
#12745=ORIENTED_EDGE ( 'NONE', *, *, #19968, .F. ) ;
#12749=CARTESIAN_POINT ( 'NONE',  ( -16.62779268661489951, 10.00000000000000000, 1.000000000000000000 ) ) ;
#12750=EDGE_LOOP ( 'NONE', ( #1963, #994, #12745, #5393 ) ) ;
#12757=CARTESIAN_POINT ( 'NONE',  ( -20.00349085826861995, 0.000000000000000000, 1.000000000000000000 ) ) ;
#12771=VERTEX_POINT ( 'NONE', #3767 ) ;
#12773=CARTESIAN_POINT ( 'NONE',  ( 28.94203811574921659, 16.00000000000000000, 1.000000000000000000 ) ) ;
#12778=CARTESIAN_POINT ( 'NONE',  ( -0.000000000000000000, 11.64110105645932691, 0.000000000000000000 ) ) ;
#12779=VECTOR ( 'NONE', #15501, 1000.000000000000000 ) ;
#12788=DIRECTION ( 'NONE',  ( 0.000000000000000000, 0.000000000000000000, -1.000000000000000000 ) ) ;
#12795=LINE ( 'NONE', #9557, #6008 ) ;
#12800=DIRECTION ( 'NONE',  ( -1.734723475976787570E-15, 1.000000000000000000, 0.000000000000000000 ) ) ;
#12803=ADVANCED_FACE ( 'NONE', ( #425 ), #8171, .T. ) ;
#12806=DIRECTION ( 'NONE',  ( 1.000000000000000000, -0.000000000000000000, 0.000000000000000000 ) ) ;
#12809=CARTESIAN_POINT ( 'NONE',  ( -15.00000000000000000, 0.000000000000000000, 1.000000000000000000 ) ) ;
#12810=LINE ( 'NONE', #3401, #19406 ) ;
#12822=VERTEX_POINT ( 'NONE', #8575 ) ;
#12831=CARTESIAN_POINT ( 'NONE',  ( -0.000000000000000000, 10.00000000000000000, 0.000000000000000000 ) ) ;
#12835=CARTESIAN_POINT ( 'NONE',  ( 0.000000000000000000, 16.00000000000000000, 1.000000000000000000 ) ) ;
#12837=VERTEX_POINT ( 'NONE', #12964 ) ;
#12844=DIRECTION ( 'NONE',  ( -0.000000000000000000, -0.000000000000000000, -1.000000000000000000 ) ) ;
#12845=ADVANCED_FACE ( 'NONE', ( #8681 ), #17036, .T. ) ;
#12846=ORIENTED_EDGE ( 'NONE', *, *, #15141, .T. ) ;
#12847=DIRECTION ( 'NONE',  ( 0.000000000000000000, 0.000000000000000000, 1.000000000000000000 ) ) ;
#12849=ORIENTED_EDGE ( 'NONE', *, *, #8607, .F. ) ;
#12854=DIRECTION ( 'NONE',  ( 0.000000000000000000, 1.000000000000000000, -0.000000000000000000 ) ) ;
#12857=DIRECTION ( 'NONE',  ( -0.000000000000000000, -0.000000000000000000, -1.000000000000000000 ) ) ;
#12868=ORIENTED_EDGE ( 'NONE', *, *, #9328, .T. ) ;
#12871=CARTESIAN_POINT ( 'NONE',  ( 0.000000000000000000, 11.64110105645932691, 10.00000000000000000 ) ) ;
#12872=CARTESIAN_POINT ( 'NONE',  ( -10.43924542913431175, 10.00000000000000000, 1.000000000000000000 ) ) ;
#12876=CARTESIAN_POINT ( 'NONE',  ( -5.563547257480587760, 11.64110105645932691, 10.00000000000000000 ) ) ;
#12879=DIRECTION ( 'NONE',  ( -1.000000000000000000, 0.000000000000000000, 0.000000000000000000 ) ) ;
#12896=EDGE_LOOP ( 'NONE', ( #9945, #8852, #7508, #17014 ) ) ;
#12899=DIRECTION ( 'NONE',  ( 0.000000000000000000, 1.000000000000000000, 0.000000000000000000 ) ) ;
#12900=LINE ( 'NONE', #12496, #3642 ) ;
#12901=CYLINDRICAL_SURFACE ( 'NONE', #7662, 10.00000000000000000 ) ;
#12903=DIRECTION ( 'NONE',  ( 0.000000000000000000, -1.000000000000000000, 0.000000000000000000 ) ) ;
#12905=LINE ( 'NONE', #1731, #4752 ) ;
#12917=DIRECTION ( 'NONE',  ( 1.000000000000000000, 0.000000000000000000, 0.000000000000000000 ) ) ;
#12918=ORIENTED_EDGE ( 'NONE', *, *, #19128, .F. ) ;
#12920=ORIENTED_EDGE ( 'NONE', *, *, #8864, .T. ) ;
#12923=LINE ( 'NONE', #14596, #11428 ) ;
#12924=VECTOR ( 'NONE', #17157, 1000.000000000000000 ) ;
#12931=EDGE_CURVE ( 'NONE', #11608, #12110, #14615, .T. ) ;
#12934=DIRECTION ( 'NONE',  ( -1.000000000000000000, 0.000000000000000000, -0.000000000000000000 ) ) ;
#12936=ORIENTED_EDGE ( 'NONE', *, *, #18887, .F. ) ;
#12941=ORIENTED_EDGE ( 'NONE', *, *, #12607, .F. ) ;
#12943=DIRECTION ( 'NONE',  ( 1.000000000000000000, -0.000000000000000000, 0.000000000000000000 ) ) ;
#12946=ORIENTED_EDGE ( 'NONE', *, *, #16692, .T. ) ;
#12950=CARTESIAN_POINT ( 'NONE',  ( -15.87779268661489773, 11.64110105645932691, 10.00000000000000000 ) ) ;
#12954=MECHANICAL_DESIGN_GEOMETRIC_PRESENTATION_REPRESENTATION('',(#7955),#4959);
#12957=VECTOR ( 'NONE', #20276, 1000.000000000000000 ) ;
#12958=ADVANCED_FACE ( 'NONE', ( #4897 ), #9713, .T. ) ;
#12960=CARTESIAN_POINT ( 'NONE',  ( 1.937849085826861328, 11.64110105645932691, 10.00000000000000000 ) ) ;
#12964=CARTESIAN_POINT ( 'NONE',  ( 26.69203811574920238, 10.00000000000000000, 0.000000000000000000 ) ) ;
#12966=VECTOR ( 'NONE', #16918, 1000.000000000000000 ) ;
#12971=ORIENTED_EDGE ( 'NONE', *, *, #6332, .F. ) ;
#12973=DIRECTION ( 'NONE',  ( 0.000000000000000000, 1.000000000000000000, 0.000000000000000000 ) ) ;
#12974=DIRECTION ( 'NONE',  ( 0.000000000000000000, 0.000000000000000000, -1.000000000000000000 ) ) ;
#12975=EDGE_LOOP ( 'NONE', ( #16891, #9272, #7962, #1563 ) ) ;
#12976=EDGE_CURVE ( 'NONE', #193, #14057, #1767, .T. ) ;
#12982=DIRECTION ( 'NONE',  ( 1.000000000000000000, 0.000000000000000000, 0.000000000000000000 ) ) ;
#12984=ADVANCED_FACE ( 'NONE', ( #9916 ), #8250, .T. ) ;
#12987=PLANE ( 'NONE',  #18758 ) ;
#12990=DIRECTION ( 'NONE',  ( 0.000000000000000000, 1.000000000000000000, 0.000000000000000000 ) ) ;
#12998=VERTEX_POINT ( 'NONE', #14517 ) ;
#13001=VECTOR ( 'NONE', #14789, 1000.000000000000000 ) ;
#13002=AXIS2_PLACEMENT_3D ( 'NONE', #13756, #7494, #4039 ) ;
#13003=DIRECTION ( 'NONE',  ( 1.000000000000000000, 0.000000000000000000, -0.000000000000000000 ) ) ;
#13004=VERTEX_POINT ( 'NONE', #8460 ) ;
#13006=VECTOR ( 'NONE', #13562, 1000.000000000000000 ) ;
#13007=ORIENTED_EDGE ( 'NONE', *, *, #1682, .T. ) ;
#13011=DIRECTION ( 'NONE',  ( 0.000000000000000000, 0.000000000000000000, -1.000000000000000000 ) ) ;
#13014=LINE ( 'NONE', #19107, #1416 ) ;
#13016=CIRCLE ( 'NONE', #3658, 10.00000000000000000 ) ;
#13020=ORIENTED_EDGE ( 'NONE', *, *, #7199, .T. ) ;
#13029=ORIENTED_EDGE ( 'NONE', *, *, #15607, .F. ) ;
#13030=ADVANCED_FACE ( 'NONE', ( #194 ), #3438, .T. ) ;
#13031=LINE ( 'NONE', #4877, #17403 ) ;
#13032=ORIENTED_EDGE ( 'NONE', *, *, #8984, .T. ) ;
#13033=CARTESIAN_POINT ( 'NONE',  ( 23.31633994409548549, 10.00000000000000000, 0.000000000000000000 ) ) ;
#13034=ADVANCED_FACE ( 'NONE', ( #13358 ), #16499, .T. ) ;
#13037=CARTESIAN_POINT ( 'NONE',  ( -13.81494360078803396, 16.00000000000000000, 1.000000000000000000 ) ) ;
#13043=SURFACE_STYLE_FILL_AREA ( #283 ) ;
#13054=DIRECTION ( 'NONE',  ( 0.000000000000000000, -0.000000000000000000, 1.000000000000000000 ) ) ;
#13055=CARTESIAN_POINT ( 'NONE',  ( -24.12918902992234393, 10.00000000000000000, 1.000000000000000000 ) ) ;
#13057=VERTEX_POINT ( 'NONE', #5001 ) ;
#13058=ORIENTED_EDGE ( 'NONE', *, *, #1948, .T. ) ;
#13060=CARTESIAN_POINT ( 'NONE',  ( 26.69203811574920238, 11.64110105645932691, 10.00000000000000000 ) ) ;
#13065=CARTESIAN_POINT ( 'NONE',  ( -0.000000000000000000, 11.64110105645932691, 0.000000000000000000 ) ) ;
#13067=AXIS2_PLACEMENT_3D ( 'NONE', #19497, #16239, #13094 ) ;
#13075=DIRECTION ( 'NONE',  ( 1.000000000000000000, 0.000000000000000000, 0.000000000000000000 ) ) ;
#13081=LINE ( 'NONE', #14854, #9438 ) ;
#13082=SURFACE_SIDE_STYLE ('',( #3564 ) ) ;
#13083=VERTEX_POINT ( 'NONE', #6683 ) ;
#13084=VECTOR ( 'NONE', #7498, 1000.000000000000000 ) ;
#13086=ORIENTED_EDGE ( 'NONE', *, *, #10682, .F. ) ;
#13088=DIRECTION ( 'NONE',  ( 1.000000000000000000, -0.000000000000000000, 0.000000000000000000 ) ) ;
#13090=LINE ( 'NONE', #14163, #15864 ) ;
#13094=DIRECTION ( 'NONE',  ( -0.000000000000000000, 0.000000000000000000, -1.000000000000000000 ) ) ;
#13098=ORIENTED_EDGE ( 'NONE', *, *, #9328, .F. ) ;
#13103=EDGE_LOOP ( 'NONE', ( #4364, #6211, #16122, #5517 ) ) ;
#13106=DIRECTION ( 'NONE',  ( -0.000000000000000000, 0.000000000000000000, -1.000000000000000000 ) ) ;
#13113=AXIS2_PLACEMENT_3D ( 'NONE', #18341, #15089, #13518 ) ;
#13119=DIRECTION ( 'NONE',  ( -1.000000000000000000, 0.000000000000000000, 0.000000000000000000 ) ) ;
#13121=EDGE_CURVE ( 'NONE', #8657, #17919, #6882, .T. ) ;
#13126=ORIENTED_EDGE ( 'NONE', *, *, #8695, .T. ) ;
#13133=CARTESIAN_POINT ( 'NONE',  ( 4.000698171653723101, 16.00000000000000000, 1.000000000000000000 ) ) ;
#13136=DIRECTION ( 'NONE',  ( 0.000000000000000000, -1.000000000000000000, 0.000000000000000000 ) ) ;
#13139=VECTOR ( 'NONE', #10781, 1000.000000000000000 ) ;
#13145=FACE_OUTER_BOUND ( 'NONE', #15238, .T. ) ;
#13146=EDGE_CURVE ( 'NONE', #6320, #3742, #10621, .T. ) ;
#13147=( NAMED_UNIT ( * ) PLANE_ANGLE_UNIT ( ) SI_UNIT ( $, .RADIAN. ) );
#13157=CARTESIAN_POINT ( 'NONE',  ( 0.000000000000000000, 16.00000000000000000, 1.000000000000000000 ) ) ;
#13161=DIRECTION ( 'NONE',  ( -1.000000000000000000, -5.782411586589356653E-16, 0.000000000000000000 ) ) ;
#13163=FACE_OUTER_BOUND ( 'NONE', #17915, .T. ) ;
#13165=DIRECTION ( 'NONE',  ( -1.000000000000000000, 0.000000000000000000, 0.000000000000000000 ) ) ;
#13174=LINE ( 'NONE', #11604, #20116 ) ;
#13178=VERTEX_POINT ( 'NONE', #712 ) ;
#13183=( NAMED_UNIT ( * ) PLANE_ANGLE_UNIT ( ) SI_UNIT ( $, .RADIAN. ) );
#13186=DIRECTION ( 'NONE',  ( 0.000000000000000000, 0.000000000000000000, -1.000000000000000000 ) ) ;
#13208=VECTOR ( 'NONE', #5794, 1000.000000000000000 ) ;
#13210=LINE ( 'NONE', #663, #9638 ) ;
#13211=CARTESIAN_POINT ( 'NONE',  ( 25.37918902992234393, 10.00000000000000000, 1.000000000000000000 ) ) ;
#13213=DIRECTION ( 'NONE',  ( -1.000000000000000000, 0.000000000000000000, 0.000000000000000000 ) ) ;
#13220=ORIENTED_EDGE ( 'NONE', *, *, #3410, .F. ) ;
#13221=VECTOR ( 'NONE', #19858, 1000.000000000000000 ) ;
#13225=ORIENTED_EDGE ( 'NONE', *, *, #7013, .F. ) ;
#13229=VERTEX_POINT ( 'NONE', #13875 ) ;
#13233=( BOUNDED_CURVE ( )  B_SPLINE_CURVE ( 3, ( #7963, #20, #6408, #12773 ),
 .UNSPECIFIED., .F., .F. ) 
 B_SPLINE_CURVE_WITH_KNOTS ( ( 4, 4 ),
 ( 4.712388980384689674, 5.163415792180952479 ),
 .UNSPECIFIED. ) 
 CURVE ( )  GEOMETRIC_REPRESENTATION_ITEM ( )  RATIONAL_B_SPLINE_CURVE ( ( 1.000000000000000000, 0.9831196229872640746, 0.9831196229872640746, 1.000000000000000000 ) ) 
 REPRESENTATION_ITEM ( '' )  );
#13236=CARTESIAN_POINT ( 'NONE',  ( -2.187849085826861550, 0.000000000000000000, 1.000000000000000000 ) ) ;
#13240=EDGE_CURVE ( 'NONE', #16093, #18054, #12205, .T. ) ;
#13247=ORIENTED_EDGE ( 'NONE', *, *, #14763, .F. ) ;
#13250=VERTEX_POINT ( 'NONE', #2380 ) ;
#13251=AXIS2_PLACEMENT_3D ( 'NONE', #14983, #3700, #3904 ) ;
#13253=CARTESIAN_POINT ( 'NONE',  ( -24.87918902992234393, 0.000000000000000000, 1.000000000000000000 ) ) ;
#13257=EDGE_CURVE ( 'NONE', #4699, #11113, #10332, .T. ) ;
#13263=LINE ( 'NONE', #10032, #4792 ) ;
#13269=DIRECTION ( 'NONE',  ( -0.000000000000000000, 0.000000000000000000, -1.000000000000000000 ) ) ;
#13270=DIRECTION ( 'NONE',  ( -0.000000000000000000, 0.000000000000000000, -1.000000000000000000 ) ) ;
#13274=ORIENTED_EDGE ( 'NONE', *, *, #7939, .F. ) ;
#13277=( LENGTH_UNIT ( ) NAMED_UNIT ( * ) SI_UNIT ( .MILLI., .METRE. ) );
#13280=CARTESIAN_POINT ( 'NONE',  ( 0.000000000000000000, 10.00000000000000000, 1.000000000000000000 ) ) ;
#13281=AXIS2_PLACEMENT_3D ( 'NONE', #3637, #14925, #16296 ) ;
#13285=AXIS2_PLACEMENT_3D ( 'NONE', #7493, #12394, #12287 ) ;
#13293=AXIS2_PLACEMENT_3D ( 'NONE', #12293, #6031, #12094 ) ;
#13303=ORIENTED_EDGE ( 'NONE', *, *, #9648, .F. ) ;
#13304=DIRECTION ( 'NONE',  ( -0.000000000000000000, -0.000000000000000000, -1.000000000000000000 ) ) ;
#13305=VECTOR ( 'NONE', #10395, 1000.000000000000114 ) ;
#13307=EDGE_CURVE ( 'NONE', #12487, #1742, #8769, .T. ) ;
#13309=VECTOR ( 'NONE', #8834, 1000.000000000000000 ) ;
#13312=EDGE_CURVE ( 'NONE', #4104, #20490, #815, .T. ) ;
#13317=CARTESIAN_POINT ( 'NONE',  ( -0.000000000000000000, 10.00000000000000000, 0.000000000000000000 ) ) ;
#13321=AXIS2_PLACEMENT_3D ( 'NONE', #13473, #18404, #725 ) ;
#13323=CIRCLE ( 'NONE', #15999, 10.00000000000000000 ) ;
#13333=VECTOR ( 'NONE', #2562, 1000.000000000000000 ) ;
#13336=ORIENTED_EDGE ( 'NONE', *, *, #3802, .T. ) ;
#13339=VERTEX_POINT ( 'NONE', #5624 ) ;
#13343=VECTOR ( 'NONE', #18338, 1000.000000000000000 ) ;
#13357=ORIENTED_EDGE ( 'NONE', *, *, #6332, .T. ) ;
#13358=FACE_OUTER_BOUND ( 'NONE', #2782, .T. ) ;
#13361=ORIENTED_EDGE ( 'NONE', *, *, #11213, .F. ) ;
#13362=EDGE_CURVE ( 'NONE', #11847, #12998, #5837, .T. ) ;
#13364=EDGE_CURVE ( 'NONE', #11847, #18960, #9080, .T. ) ;
#13365=ORIENTED_EDGE ( 'NONE', *, *, #9150, .F. ) ;
#13376=EDGE_CURVE ( 'NONE', #13004, #1633, #9381, .T. ) ;
#13378=VECTOR ( 'NONE', #17189, 1000.000000000000000 ) ;
#13379=VECTOR ( 'NONE', #19943, 1000.000000000000000 ) ;
#13385=VERTEX_POINT ( 'NONE', #10955 ) ;
#13387=CARTESIAN_POINT ( 'NONE',  ( 0.000000000000000000, 10.00000000000000000, 1.000000000000000000 ) ) ;
#13390=AXIS2_PLACEMENT_3D ( 'NONE', #4917, #9523, #19265 ) ;
#13395=AXIS2_PLACEMENT_3D ( 'NONE', #14555, #3373, #10912 ) ;
#13396=DIRECTION ( 'NONE',  ( 0.000000000000000000, 0.000000000000000000, -1.000000000000000000 ) ) ;
#13398=CARTESIAN_POINT ( 'NONE',  ( 17.12779268661489596, 10.00000000000000000, 0.000000000000000000 ) ) ;
#13406=CIRCLE ( 'NONE', #4403, 10.00000000000000000 ) ;
#13409=ORIENTED_EDGE ( 'NONE', *, *, #10847, .T. ) ;
#13415=CARTESIAN_POINT ( 'NONE',  ( -17.94064177244175795, 10.00000000000000000, 1.000000000000000000 ) ) ;
#13418=CIRCLE ( 'NONE', #5764, 2.999999999999999112 ) ;
#13419=DIRECTION ( 'NONE',  ( 0.000000000000000000, 1.000000000000000000, -0.000000000000000000 ) ) ;
#13421=PLANE ( 'NONE',  #2368 ) ;
#13422=LINE ( 'NONE', #5377, #19086 ) ;
#13433=ORIENTED_EDGE ( 'NONE', *, *, #5064, .T. ) ;
#13436=ORIENTED_EDGE ( 'NONE', *, *, #6466, .T. ) ;
#13438=AXIS2_PLACEMENT_3D ( 'NONE', #6434, #12800, #19200 ) ;
#13439=LINE ( 'NONE', #12081, #13379 ) ;
#13443=ADVANCED_FACE ( 'NONE', ( #18809 ), #4670, .T. ) ;
#13444=ORIENTED_EDGE ( 'NONE', *, *, #15750, .T. ) ;
#13454=CARTESIAN_POINT ( 'NONE',  ( -12.50209451496117197, 10.00000000000000000, 1.000000000000000000 ) ) ;
#13456=ADVANCED_FACE ( 'NONE', ( #6044 ), #20588, .T. ) ;
#13458=ORIENTED_EDGE ( 'NONE', *, *, #18197, .T. ) ;
#13463=DIRECTION ( 'NONE',  ( -1.000000000000000000, 0.000000000000000000, 0.000000000000000000 ) ) ;
#13466=VECTOR ( 'NONE', #6019, 1000.000000000000000 ) ;
#13470=CARTESIAN_POINT ( 'NONE',  ( -11.75209451496117197, 10.00000000000000000, 1.000000000000000000 ) ) ;
#13473=CARTESIAN_POINT ( 'NONE',  ( 6.813547257480585095, 0.000000000000000000, 1.000000000000000000 ) ) ;
#13476=CARTESIAN_POINT ( 'NONE',  ( -12.50209451496117197, 0.000000000000000000, 1.000000000000000000 ) ) ;
#13481=VERTEX_POINT ( 'NONE', #9277 ) ;
#13483=DIRECTION ( 'NONE',  ( 0.000000000000000000, 0.000000000000000000, 1.000000000000000000 ) ) ;
#13489=VERTEX_POINT ( 'NONE', #13975 ) ;
#13497=EDGE_CURVE ( 'NONE', #17944, #12390, #7298, .T. ) ;
#13504=CARTESIAN_POINT ( 'NONE',  ( 25.37918902992234393, 11.64110105645932691, 0.000000000000000000 ) ) ;
#13512=ORIENTED_EDGE ( 'NONE', *, *, #2983, .F. ) ;
#13518=DIRECTION ( 'NONE',  ( 1.000000000000000000, 0.000000000000000000, 0.000000000000000000 ) ) ;
#13519=EDGE_CURVE ( 'NONE', #14797, #9402, #2901, .T. ) ;
#13520=CYLINDRICAL_SURFACE ( 'NONE', #13251, 10.00000000000000000 ) ;
#13521=CARTESIAN_POINT ( 'NONE',  ( 12.25209451496117197, 0.000000000000000000, 0.000000000000000000 ) ) ;
#13522=LINE ( 'NONE', #19924, #13001 ) ;
#13524=DIRECTION ( 'NONE',  ( 0.000000000000000000, 0.000000000000000000, 1.000000000000000000 ) ) ;
#13535=VERTEX_POINT ( 'NONE', #7915 ) ;
#13538=VERTEX_POINT ( 'NONE', #1337 ) ;
#13541=CARTESIAN_POINT ( 'NONE',  ( 23.31633994409548549, 16.00000000000000000, 1.000000000000000000 ) ) ;
#13545=PLANE ( 'NONE',  #7535 ) ;
#13557=ORIENTED_EDGE ( 'NONE', *, *, #2620, .T. ) ;
#13562=DIRECTION ( 'NONE',  ( 0.000000000000000000, -1.000000000000000000, 0.000000000000000000 ) ) ;
#13567=LINE ( 'NONE', #12006, #7967 ) ;
#13571=LINE ( 'NONE', #2184, #11805 ) ;
#13573=EDGE_CURVE ( 'NONE', #3633, #13083, #15856, .T. ) ;
#13574=EDGE_CURVE ( 'NONE', #4233, #7302, #12720, .T. ) ;
#13578=EDGE_LOOP ( 'NONE', ( #13800, #18522, #8014, #7785 ) ) ;
#13579=DIRECTION ( 'NONE',  ( 0.000000000000000000, 0.000000000000000000, 1.000000000000000000 ) ) ;
#13582=EDGE_CURVE ( 'NONE', #1441, #14649, #2152, .T. ) ;
#13586=ORIENTED_EDGE ( 'NONE', *, *, #11698, .T. ) ;
#13590=LINE ( 'NONE', #4188, #9461 ) ;
#13591=CIRCLE ( 'NONE', #2581, 10.00000000000000000 ) ;
#13592=CARTESIAN_POINT ( 'NONE',  ( 8.126396343307449754, 10.00000000000000000, 0.000000000000000000 ) ) ;
#13593=FACE_OUTER_BOUND ( 'NONE', #2357, .T. ) ;
#13594=DIRECTION ( 'NONE',  ( -1.000000000000000000, 0.000000000000000000, 0.000000000000000000 ) ) ;
#13595=EDGE_CURVE ( 'NONE', #11608, #20520, #13031, .T. ) ;
#13613=ORIENTED_EDGE ( 'NONE', *, *, #5016, .T. ) ;
#13614=LINE ( 'NONE', #17176, #11444 ) ;
#13615=DIRECTION ( 'NONE',  ( -1.000000000000000000, 0.000000000000000000, 0.000000000000000000 ) ) ;
#13617=EDGE_CURVE ( 'NONE', #351, #13057, #17945, .T. ) ;
#13618=DIRECTION ( 'NONE',  ( 0.000000000000000000, -1.000000000000000000, 0.000000000000000000 ) ) ;
#13622=PLANE ( 'NONE',  #711 ) ;
#13629=EDGE_CURVE ( 'NONE', #5929, #6320, #8534, .T. ) ;
#13632=ORIENTED_EDGE ( 'NONE', *, *, #18198, .F. ) ;
#13638=CARTESIAN_POINT ( 'NONE',  ( 20.50349085826861995, 0.000000000000000000, 1.000000000000000000 ) ) ;
#13644=DIRECTION ( 'NONE',  ( -0.000000000000000000, -0.000000000000000000, -1.000000000000000000 ) ) ;
#13649=AXIS2_PLACEMENT_3D ( 'NONE', #13253, #13463, #2077 ) ;
#13650=LINE ( 'NONE', #8546, #1614 ) ;
#13657=ORIENTED_EDGE ( 'NONE', *, *, #10520, .T. ) ;
#13659=FACE_OUTER_BOUND ( 'NONE', #4828, .T. ) ;
#13661=CARTESIAN_POINT ( 'NONE',  ( 17.12779268661489596, 0.000000000000000000, 0.000000000000000000 ) ) ;
#13664=AXIS2_PLACEMENT_3D ( 'NONE', #363, #8515, #6842 ) ;
#13665=ORIENTED_EDGE ( 'NONE', *, *, #20684, .T. ) ;
#13667=AXIS2_PLACEMENT_3D ( 'NONE', #7288, #4465, #10850 ) ;
#13669=CARTESIAN_POINT ( 'NONE',  ( -10.38119784648305632, -14.00000000000000000, 2.000000000000000000 ) ) ;
#13670=DIRECTION ( 'NONE',  ( 1.000000000000000000, 0.000000000000000000, 0.000000000000000000 ) ) ;
#13672=LINE ( 'NONE', #15458, #17710 ) ;
#13674=LINE ( 'NONE', #2708, #10026 ) ;
#13675=VECTOR ( 'NONE', #19283, 1000.000000000000000 ) ;
#13681=DIRECTION ( 'NONE',  ( 1.000000000000000000, 0.000000000000000000, 0.000000000000000000 ) ) ;
#13690=CARTESIAN_POINT ( 'NONE',  ( -8.376396343307449754, 10.00000000000000000, 1.000000000000000000 ) ) ;
#13696=DIRECTION ( 'NONE',  ( 0.000000000000000000, -1.000000000000000000, 0.000000000000000000 ) ) ;
#13699=AXIS2_PLACEMENT_3D ( 'NONE', #5877, #12247, #2841 ) ;
#13704=DIRECTION ( 'NONE',  ( 1.156482317317871133E-15, -1.000000000000000000, 0.000000000000000000 ) ) ;
#13713=ORIENTED_EDGE ( 'NONE', *, *, #1313, .F. ) ;
#13715=CARTESIAN_POINT ( 'NONE',  ( 1.937849085826861328, 0.000000000000000000, 1.000000000000000000 ) ) ;
#13716=VECTOR ( 'NONE', #16073, 1000.000000000000000 ) ;
#13717=ORIENTED_EDGE ( 'NONE', *, *, #8398, .F. ) ;
#13718=VECTOR ( 'NONE', #11753, 1000.000000000000000 ) ;
#13721=DIRECTION ( 'NONE',  ( 1.000000000000000000, 0.000000000000000000, 0.000000000000000000 ) ) ;
#13738=CARTESIAN_POINT ( 'NONE',  ( 13.00209451496117374, 10.00000000000000000, 1.000000000000000000 ) ) ;
#13746=VERTEX_POINT ( 'NONE', #8328 ) ;
#13749=EDGE_CURVE ( 'NONE', #346, #4104, #384, .T. ) ;
#13756=CARTESIAN_POINT ( 'NONE',  ( 10.93924542913430820, 11.64110105645932691, 10.00000000000000000 ) ) ;
#13767=AXIS2_PLACEMENT_3D ( 'NONE', #19736, #7076, #3926 ) ;
#13769=EDGE_LOOP ( 'NONE', ( #6266, #12946, #13713, #3843 ) ) ;
#13772=VERTEX_POINT ( 'NONE', #8441 ) ;
#13775=ORIENTED_EDGE ( 'NONE', *, *, #19157, .T. ) ;
#13779=FACE_OUTER_BOUND ( 'NONE', #11302, .T. ) ;
#13780=EDGE_CURVE ( 'NONE', #10885, #15705, #6862, .T. ) ;
#13781=CARTESIAN_POINT ( 'NONE',  ( -12.50209451496117197, 11.64110105645932691, 0.000000000000000000 ) ) ;
#13785=CARTESIAN_POINT ( 'NONE',  ( 27.44203811574919882, 10.00000000000000000, 1.000000000000000000 ) ) ;
#13793=CIRCLE ( 'NONE', #4782, 1.499999999999996225 ) ;
#13796=ORIENTED_EDGE ( 'NONE', *, *, #13257, .T. ) ;
#13799=DIRECTION ( 'NONE',  ( 0.000000000000000000, -1.000000000000000000, 0.000000000000000000 ) ) ;
#13800=ORIENTED_EDGE ( 'NONE', *, *, #17369, .T. ) ;
#13805=VECTOR ( 'NONE', #3650, 1000.000000000000000 ) ;
#13806=LINE ( 'NONE', #18942, #14825 ) ;
#13809=LINE ( 'NONE', #8907, #16724 ) ;
#13820=DIRECTION ( 'NONE',  ( 1.000000000000000000, 0.000000000000000000, -0.000000000000000000 ) ) ;
#13823=LINE ( 'NONE', #18650, #8777 ) ;
#13835=EDGE_CURVE ( 'NONE', #4154, #8135, #13439, .T. ) ;
#13845=EDGE_LOOP ( 'NONE', ( #2384, #221, #19199, #13336 ) ) ;
#13846=EDGE_CURVE ( 'NONE', #965, #19224, #16572, .T. ) ;
#13848=DIRECTION ( 'NONE',  ( 0.000000000000000000, 0.000000000000000000, -1.000000000000000000 ) ) ;
#13852=ORIENTED_EDGE ( 'NONE', *, *, #15273, .F. ) ;
#13854=DIRECTION ( 'NONE',  ( 0.000000000000000000, 1.000000000000000000, -0.000000000000000000 ) ) ;
#13875=CARTESIAN_POINT ( 'NONE',  ( -6.313547257480587760, 11.64110105645932691, 0.000000000000000000 ) ) ;
#13879=LINE ( 'NONE', #20185, #18345 ) ;
#13880=DIRECTION ( 'NONE',  ( 1.000000000000000000, 0.000000000000000000, 0.000000000000000000 ) ) ;
#13881=EDGE_CURVE ( 'NONE', #4496, #15932, #18370, .T. ) ;
#13884=CARTESIAN_POINT ( 'NONE',  ( -27.94203811574920948, 16.00000000000000000, 1.000000000000000000 ) ) ;
#13886=LINE ( 'NONE', #20287, #3680 ) ;
#13890=ORIENTED_EDGE ( 'NONE', *, *, #7828, .F. ) ;
#13894=VERTEX_POINT ( 'NONE', #16788 ) ;
#13895=EDGE_CURVE ( 'NONE', #175, #16502, #687, .T. ) ;
#13898=ORIENTED_EDGE ( 'NONE', *, *, #5507, .F. ) ;
#13899=VERTEX_POINT ( 'NONE', #8943 ) ;
#13903=DIRECTION ( 'NONE',  ( 1.000000000000000000, 0.000000000000000000, 0.000000000000000000 ) ) ;
#13906=DIRECTION ( 'NONE',  ( 0.000000000000000000, 0.000000000000000000, 1.000000000000000000 ) ) ;
#13927=LINE ( 'NONE', #13521, #5293 ) ;
#13929=LINE ( 'NONE', #20026, #20692 ) ;
#13932=FACE_OUTER_BOUND ( 'NONE', #12750, .T. ) ;
#13933=LINE ( 'NONE', #15202, #11316 ) ;
#13936=ORIENTED_EDGE ( 'NONE', *, *, #16387, .F. ) ;
#13937=VECTOR ( 'NONE', #18289, 1000.000000000000000 ) ;
#13939=FACE_OUTER_BOUND ( 'NONE', #15623, .T. ) ;
#13944=LINE ( 'NONE', #6118, #8714 ) ;
#13945=VERTEX_POINT ( 'NONE', #13541 ) ;
#13950=PLANE ( 'NONE',  #17444 ) ;
#13951=CARTESIAN_POINT ( 'NONE',  ( -0.000000000000000000, 10.00000000000000000, 0.000000000000000000 ) ) ;
#13953=EDGE_CURVE ( 'NONE', #19964, #8687, #996, .T. ) ;
#13956=PLANE ( 'NONE',  #16035 ) ;
#13957=AXIS2_PLACEMENT_3D ( 'NONE', #5762, #100, #20715 ) ;
#13962=CYLINDRICAL_SURFACE ( 'NONE', #18990, 2.999999999999999112 ) ;
#13965=VECTOR ( 'NONE', #5940, 1000.000000000000000 ) ;
#13970=VECTOR ( 'NONE', #19236, 1000.000000000000000 ) ;
#13973=DIRECTION ( 'NONE',  ( 1.000000000000000000, -0.000000000000000000, 0.000000000000000000 ) ) ;
#13975=CARTESIAN_POINT ( 'NONE',  ( 28.94203811574921659, 16.00000000000000000, 1.000000000000000000 ) ) ;
#13976=EDGE_CURVE ( 'NONE', #20490, #5162, #9155, .T. ) ;
#13982=VECTOR ( 'NONE', #6818, 1000.000000000000000 ) ;
#13984=PLANE ( 'NONE',  #15322 ) ;
#13985=LINE ( 'NONE', #12525, #6967 ) ;
#13986=AXIS2_PLACEMENT_3D ( 'NONE', #14837, #19656, #16506 ) ;
#13987=ADVANCED_FACE ( 'NONE', ( #9742 ), #9353, .T. ) ;
#13991=VERTEX_POINT ( 'NONE', #16014 ) ;
#13993=LINE ( 'NONE', #18929, #727 ) ;
#13997=VERTEX_POINT ( 'NONE', #10726 ) ;
#13999=EDGE_CURVE ( 'NONE', #2481, #20051, #12492, .T. ) ;
#14006=LINE ( 'NONE', #13690, #20275 ) ;
#14008=CARTESIAN_POINT ( 'NONE',  ( -8.376396343307449754, 10.00000000000000000, 1.000000000000000000 ) ) ;
#14010=DIRECTION ( 'NONE',  ( -0.000000000000000000, -0.000000000000000000, -1.000000000000000000 ) ) ;
#14018=AXIS2_PLACEMENT_3D ( 'NONE', #14269, #17519, #20578 ) ;
#14033=CIRCLE ( 'NONE', #18398, 10.00000000000000000 ) ;
#14037=EDGE_CURVE ( 'NONE', #411, #6312, #19376, .T. ) ;
#14038=DIRECTION ( 'NONE',  ( 1.000000000000000000, 0.000000000000000000, -0.000000000000000000 ) ) ;
#14039=CARTESIAN_POINT ( 'NONE',  ( 27.00000000000000000, 0.000000000000000000, 0.000000000000000000 ) ) ;
#14041=DIRECTION ( 'NONE',  ( 0.000000000000000000, 0.000000000000000000, 1.000000000000000000 ) ) ;
#14047=VECTOR ( 'NONE', #16244, 1000.000000000000000 ) ;
#14051=VECTOR ( 'NONE', #8088, 1000.000000000000000 ) ;
#14057=VERTEX_POINT ( 'NONE', #7584 ) ;
#14060=VERTEX_POINT ( 'NONE', #124 ) ;
#14067=PLANE ( 'NONE',  #1475 ) ;
#14069=EDGE_CURVE ( 'NONE', #2663, #12837, #6605, .T. ) ;
#14070=LINE ( 'NONE', #1123, #3615 ) ;
#14071=CARTESIAN_POINT ( 'NONE',  ( 20.50349085826861995, 11.64110105645932691, 10.00000000000000000 ) ) ;
#14078=ADVANCED_FACE ( 'NONE', ( #7687 ), #11304, .T. ) ;
#14087=VERTEX_POINT ( 'NONE', #12280 ) ;
#14094=ADVANCED_FACE ( 'NONE', ( #3361 ), #219, .T. ) ;
#14097=LINE ( 'NONE', #20397, #7870 ) ;
#14103=ORIENTED_EDGE ( 'NONE', *, *, #1584, .F. ) ;
#14104=AXIS2_PLACEMENT_3D ( 'NONE', #2299, #11716, #743 ) ;
#14108=CARTESIAN_POINT ( 'NONE',  ( -14.56494360078803396, 11.64110105645932691, 10.00000000000000000 ) ) ;
#14113=DIRECTION ( 'NONE',  ( 1.000000000000000000, -3.469446951953491127E-15, 0.000000000000000000 ) ) ;
#14117=FACE_OUTER_BOUND ( 'NONE', #20564, .T. ) ;
#14125=VECTOR ( 'NONE', #7692, 1000.000000000000000 ) ;
#14134=VECTOR ( 'NONE', #12854, 1000.000000000000000 ) ;
#14136=CARTESIAN_POINT ( 'NONE',  ( 0.000000000000000000, 11.64110105645932691, 10.00000000000000000 ) ) ;
#14140=ADVANCED_FACE ( 'NONE', ( #17690 ), #3463, .T. ) ;
#14141=CARTESIAN_POINT ( 'NONE',  ( 4.750698171653723989, 10.00000000000000000, 1.000000000000000000 ) ) ;
#14144=CARTESIAN_POINT ( 'NONE',  ( -10.43924542913431175, 16.00000000000000000, 1.000000000000000000 ) ) ;
#14156=DIRECTION ( 'NONE',  ( 0.000000000000000000, -1.000000000000000000, 0.000000000000000000 ) ) ;
#14160=PLANE ( 'NONE',  #20467 ) ;
#14163=CARTESIAN_POINT ( 'NONE',  ( 30.00000000000000000, 0.000000000000000000, 1.000000000000000000 ) ) ;
#14165=DIRECTION ( 'NONE',  ( 1.000000000000000000, 0.000000000000000000, 0.000000000000000000 ) ) ;
#14169=CARTESIAN_POINT ( 'NONE',  ( 8.876396343307449754, 11.64110105645932691, 0.000000000000000000 ) ) ;
#14170=PLANE ( 'NONE',  #5041 ) ;
#14171=CARTESIAN_POINT ( 'NONE',  ( 6.813547257480585095, 10.00000000000000000, 1.000000000000000000 ) ) ;
#14180=CARTESIAN_POINT ( 'NONE',  ( -9.689245429134309973, 0.000000000000000000, 0.000000000000000000 ) ) ;
#14181=ORIENTED_EDGE ( 'NONE', *, *, #15750, .F. ) ;
#14186=LINE ( 'NONE', #9696, #8304 ) ;
#14197=DIRECTION ( 'NONE',  ( 1.000000000000000000, 0.000000000000000000, 0.000000000000000000 ) ) ;
#14205=EDGE_CURVE ( 'NONE', #1368, #4668, #13081, .T. ) ;
#14207=ORIENTED_EDGE ( 'NONE', *, *, #11198, .T. ) ;
#14209=CARTESIAN_POINT ( 'NONE',  ( -0.000000000000000000, 10.00000000000000000, 0.000000000000000000 ) ) ;
#14214=LINE ( 'NONE', #18944, #660 ) ;
#14229=CARTESIAN_POINT ( 'NONE',  ( 0.000000000000000000, 16.00000000000000000, 1.000000000000000000 ) ) ;
#14230=LINE ( 'NONE', #11115, #5933 ) ;
#14234=CARTESIAN_POINT ( 'NONE',  ( 24.62918902992234038, 16.00000000000000000, 1.000000000000000000 ) ) ;
#14246=EDGE_LOOP ( 'NONE', ( #6582, #3513, #15026, #287 ) ) ;
#14253=ADVANCED_FACE ( 'NONE', ( #5341 ), #3977, .T. ) ;
#14255=CARTESIAN_POINT ( 'NONE',  ( -30.00000000000000000, 0.000000000000000000, 1.000000000000000000 ) ) ;
#14256=VECTOR ( 'NONE', #204, 1000.000000000000000 ) ;
#14257=ORIENTED_EDGE ( 'NONE', *, *, #5268, .F. ) ;
#14260=CARTESIAN_POINT ( 'NONE',  ( 0.000000000000000000, 10.00000000000000000, 1.000000000000000000 ) ) ;
#14269=CARTESIAN_POINT ( 'NONE',  ( -22.06633994409548194, 0.000000000000000000, 1.000000000000000000 ) ) ;
#14274=ORIENTED_EDGE ( 'NONE', *, *, #17834, .F. ) ;
#14276=CARTESIAN_POINT ( 'NONE',  ( 14.31494360078803041, 11.64110105645932691, 0.000000000000000000 ) ) ;
#14278=VECTOR ( 'NONE', #13880, 1000.000000000000000 ) ;
#14279=DIRECTION ( 'NONE',  ( -0.000000000000000000, -0.000000000000000000, -1.000000000000000000 ) ) ;
#14286=CARTESIAN_POINT ( 'NONE',  ( 0.000000000000000000, 10.00000000000000000, 1.000000000000000000 ) ) ;
#14290=SURFACE_STYLE_USAGE ( .BOTH. , #17445 ) ;
#14294=ORIENTED_EDGE ( 'NONE', *, *, #1366, .T. ) ;
#14302=ADVANCED_FACE ( 'NONE', ( #531 ), #14647, .T. ) ;
#14305=ORIENTED_EDGE ( 'NONE', *, *, #15540, .T. ) ;
#14308=VECTOR ( 'NONE', #2807, 1000.000000000000000 ) ;
#14309=EDGE_LOOP ( 'NONE', ( #2874, #388, #2558, #3951 ) ) ;
#14310=CIRCLE ( 'NONE', #9647, 1.499999999999996225 ) ;
#14313=CARTESIAN_POINT ( 'NONE',  ( 4.000698171653723101, 0.000000000000000000, 1.000000000000000000 ) ) ;
#14315=VECTOR ( 'NONE', #3218, 1000.000000000000000 ) ;
#14318=AXIS2_PLACEMENT_3D ( 'NONE', #8421, #3807, #6941 ) ;
#14321=EDGE_CURVE ( 'NONE', #7216, #20520, #6146, .T. ) ;
#14337=DIRECTION ( 'NONE',  ( 1.000000000000000000, 0.000000000000000000, -0.000000000000000000 ) ) ;
#14339=AXIS2_PLACEMENT_3D ( 'NONE', #3695, #13003, #13106 ) ;
#14340=AXIS2_PLACEMENT_3D ( 'NONE', #6033, #12405, #18799 ) ;
#14349=EDGE_CURVE ( 'NONE', #10513, #13481, #7020, .T. ) ;
#14353=CARTESIAN_POINT ( 'NONE',  ( 24.62918902992234038, 0.000000000000000000, 1.000000000000000000 ) ) ;
#14362=AXIS2_PLACEMENT_3D ( 'NONE', #5039, #14337, #19279 ) ;
#14364=FACE_OUTER_BOUND ( 'NONE', #12896, .T. ) ;
#14366=CARTESIAN_POINT ( 'NONE',  ( 0.000000000000000000, 10.00000000000000000, 1.000000000000000000 ) ) ;
#14367=DIRECTION ( 'NONE',  ( -1.000000000000000000, 0.000000000000000000, 0.000000000000000000 ) ) ;
#14377=CARTESIAN_POINT ( 'NONE',  ( -14.56494360078803396, 0.000000000000000000, 1.000000000000000000 ) ) ;
#14380=LINE ( 'NONE', #14171, #20387 ) ;
#14388=ORIENTED_EDGE ( 'NONE', *, *, #1872, .T. ) ;
#14389=ORIENTED_EDGE ( 'NONE', *, *, #3250, .T. ) ;
#14394=EDGE_CURVE ( 'NONE', #8920, #682, #10883, .T. ) ;
#14395=VECTOR ( 'NONE', #12675, 999.9999999999998863 ) ;
#14397=ORIENTED_EDGE ( 'NONE', *, *, #7601, .F. ) ;
#14404=FACE_BOUND ( 'NONE', #2692, .T. ) ;
#14406=AXIS2_PLACEMENT_3D ( 'NONE', #2649, #20334, #7471 ) ;
#14407=ORIENTED_EDGE ( 'NONE', *, *, #18571, .F. ) ;
#14431=VECTOR ( 'NONE', #20350, 1000.000000000000000 ) ;
#14436=CIRCLE ( 'NONE', #10764, 10.00000000000000000 ) ;
#14442=DIRECTION ( 'NONE',  ( 0.000000000000000000, -0.000000000000000000, 1.000000000000000000 ) ) ;
#14444=ORIENTED_EDGE ( 'NONE', *, *, #11899, .F. ) ;
#14446=DIRECTION ( 'NONE',  ( 0.000000000000000000, 1.000000000000000000, -0.000000000000000000 ) ) ;
#14451=VECTOR ( 'NONE', #13721, 1000.000000000000000 ) ;
#14452=EDGE_CURVE ( 'NONE', #6116, #17844, #2723, .T. ) ;
#14473=CARTESIAN_POINT ( 'NONE',  ( -20.75349085826862350, 0.000000000000000000, 0.000000000000000000 ) ) ;
#14475=CARTESIAN_POINT ( 'NONE',  ( 22.56633994409548194, 11.64110105645932691, 10.00000000000000000 ) ) ;
#14477=EDGE_CURVE ( 'NONE', #7631, #16888, #14006, .T. ) ;
#14493=CARTESIAN_POINT ( 'NONE',  ( 18.44064177244175440, 10.00000000000000000, 1.000000000000000000 ) ) ;
#14495=ORIENTED_EDGE ( 'NONE', *, *, #1584, .T. ) ;
#14500=ORIENTED_EDGE ( 'NONE', *, *, #1338, .T. ) ;
#14502=DIRECTION ( 'NONE',  ( 1.000000000000000000, 0.000000000000000000, 0.000000000000000000 ) ) ;
#14507=EDGE_CURVE ( 'NONE', #12054, #11489, #18525, .T. ) ;
#14509=CARTESIAN_POINT ( 'NONE',  ( 0.000000000000000000, 0.000000000000000000, 2.000000000000000000 ) ) ;
#14517=CARTESIAN_POINT ( 'NONE',  ( -6.313547257480587760, 10.00000000000000000, 0.000000000000000000 ) ) ;
#14520=PRODUCT_DEFINITION_SHAPE ( 'NONE', 'NONE',  #15961 ) ;
#14522=VERTEX_POINT ( 'NONE', #9001 ) ;
#14524=DIRECTION ( 'NONE',  ( -1.000000000000000000, 0.000000000000000000, -0.000000000000000000 ) ) ;
#14529=LINE ( 'NONE', #14209, #4580 ) ;
#14537=EDGE_CURVE ( 'NONE', #4233, #13991, #12336, .T. ) ;
#14538=DIRECTION ( 'NONE',  ( -0.000000000000000000, 0.000000000000000000, 1.000000000000000000 ) ) ;
#14544=ORIENTED_EDGE ( 'NONE', *, *, #4493, .T. ) ;
#14555=CARTESIAN_POINT ( 'NONE',  ( -24.87918902992234393, 11.64110105645932691, 10.00000000000000000 ) ) ;
#14573=DIRECTION ( 'NONE',  ( -0.000000000000000000, -0.000000000000000000, -1.000000000000000000 ) ) ;
#14574=LINE ( 'NONE', #15934, #555 ) ;
#14579=DIRECTION ( 'NONE',  ( 0.000000000000000000, 0.000000000000000000, 1.000000000000000000 ) ) ;
#14587=ADVANCED_FACE ( 'NONE', ( #10471 ), #16838, .F. ) ;
#14592=ORIENTED_EDGE ( 'NONE', *, *, #5687, .T. ) ;
#14593=ORIENTED_EDGE ( 'NONE', *, *, #972, .F. ) ;
#14594=CARTESIAN_POINT ( 'NONE',  ( 21.25349085826861995, 0.000000000000000000, 1.000000000000000000 ) ) ;
#14596=CARTESIAN_POINT ( 'NONE',  ( 0.000000000000000000, 10.00000000000000000, 1.000000000000000000 ) ) ;
#14597=EDGE_CURVE ( 'NONE', #1770, #2917, #15984, .T. ) ;
#14603=DIRECTION ( 'NONE',  ( 1.000000000000000000, 0.000000000000000000, 0.000000000000000000 ) ) ;
#14615=CIRCLE ( 'NONE', #5605, 10.00000000000000000 ) ;
#14620=VERTEX_POINT ( 'NONE', #1462 ) ;
#14621=CARTESIAN_POINT ( 'NONE',  ( 8.126396343307449754, 16.00000000000000000, 1.000000000000000000 ) ) ;
#14622=ORIENTED_EDGE ( 'NONE', *, *, #16412, .T. ) ;
#14626=VECTOR ( 'NONE', #17646, 1000.000000000000000 ) ;
#14637=CARTESIAN_POINT ( 'NONE',  ( -0.1250000000000001110, 10.00000000000000000, 0.000000000000000000 ) ) ;
#14639=VECTOR ( 'NONE', #20186, 1000.000000000000000 ) ;
#14642=VECTOR ( 'NONE', #5660, 1000.000000000000000 ) ;
#14643=ORIENTED_EDGE ( 'NONE', *, *, #8340, .F. ) ;
#14645=ORIENTED_EDGE ( 'NONE', *, *, #12135, .T. ) ;
#14647=PLANE ( 'NONE',  #3466 ) ;
#14649=VERTEX_POINT ( 'NONE', #17558 ) ;
#14655=AXIS2_PLACEMENT_3D ( 'NONE', #6939, #2133, #8514 ) ;
#14656=LINE ( 'NONE', #11421, #2504 ) ;
#14666=EDGE_LOOP ( 'NONE', ( #13613, #7833, #5186, #14803, #5949 ) ) ;
#14674=AXIS2_PLACEMENT_3D ( 'NONE', #9136, #10596, #1188 ) ;
#14675=CARTESIAN_POINT ( 'NONE',  ( 17.12779268661489596, 0.000000000000000000, 1.000000000000000000 ) ) ;
#14676=ORIENTED_EDGE ( 'NONE', *, *, #13121, .T. ) ;
#14677=AXIS2_PLACEMENT_3D ( 'NONE', #6741, #3586, #9966 ) ;
#14678=ORIENTED_EDGE ( 'NONE', *, *, #15141, .F. ) ;
#14679=CARTESIAN_POINT ( 'NONE',  ( -27.00000000000000000, 0.000000000000000000, 1.000000000000000000 ) ) ;
#14680=EDGE_CURVE ( 'NONE', #9626, #20665, #3334, .T. ) ;
#14682=DIRECTION ( 'NONE',  ( 0.000000000000000000, 1.000000000000000000, -0.000000000000000000 ) ) ;
#14685=LINE ( 'NONE', #19612, #6393 ) ;
#14692=ORIENTED_EDGE ( 'NONE', *, *, #1174, .T. ) ;
#14695=VECTOR ( 'NONE', #2284, 1000.000000000000000 ) ;
#14697=ORIENTED_EDGE ( 'NONE', *, *, #4062, .F. ) ;
#14701=ORIENTED_EDGE ( 'NONE', *, *, #14872, .T. ) ;
#14712=VECTOR ( 'NONE', #11614, 1000.000000000000000 ) ;
#14721=VERTEX_POINT ( 'NONE', #4591 ) ;
#14725=AXIS2_PLACEMENT_3D ( 'NONE', #18104, #8478, #2094 ) ;
#14727=VECTOR ( 'NONE', #5707, 1000.000000000000000 ) ;
#14728=VECTOR ( 'NONE', #4741, 1000.000000000000000 ) ;
#14730=DIRECTION ( 'NONE',  ( 1.000000000000000000, 0.000000000000000000, 0.000000000000000000 ) ) ;
#14735=DIRECTION ( 'NONE',  ( 1.000000000000000000, 0.000000000000000000, -0.000000000000000000 ) ) ;
#14737=CARTESIAN_POINT ( 'NONE',  ( 0.000000000000000000, 16.00000000000000000, 1.000000000000000000 ) ) ;
#14739=EDGE_CURVE ( 'NONE', #18649, #2409, #18963, .T. ) ;
#14741=VECTOR ( 'NONE', #19078, 1000.000000000000000 ) ;
#14753=VERTEX_POINT ( 'NONE', #4900 ) ;
#14756=CARTESIAN_POINT ( 'NONE',  ( -17.94064177244175795, 16.00000000000000000, 1.000000000000000000 ) ) ;
#14757=VERTEX_POINT ( 'NONE', #17660 ) ;
#14758=VECTOR ( 'NONE', #12326, 1000.000000000000000 ) ;
#14763=EDGE_CURVE ( 'NONE', #15727, #8843, #3648, .T. ) ;
#14773=CARTESIAN_POINT ( 'NONE',  ( 21.25349085826861995, 0.000000000000000000, 1.000000000000000000 ) ) ;
#14774=EDGE_CURVE ( 'NONE', #13772, #10231, #10276, .T. ) ;
#14781=VERTEX_POINT ( 'NONE', #13470 ) ;
#14782=ORIENTED_EDGE ( 'NONE', *, *, #18958, .T. ) ;
#14784=AXIS2_PLACEMENT_3D ( 'NONE', #1898, #14856, #16528 ) ;
#14786=EDGE_CURVE ( 'NONE', #13894, #13945, #6259, .T. ) ;
#14787=ADVANCED_FACE ( 'NONE', ( #13163 ), #10030, .F. ) ;
#14789=DIRECTION ( 'NONE',  ( 0.000000000000000000, -1.000000000000000000, 0.000000000000000000 ) ) ;
#14794=LINE ( 'NONE', #16363, #5296 ) ;
#14797=VERTEX_POINT ( 'NONE', #2386 ) ;
#14800=VECTOR ( 'NONE', #14113, 1000.000000000000000 ) ;
#14803=ORIENTED_EDGE ( 'NONE', *, *, #18103, .F. ) ;
#14818=DIRECTION ( 'NONE',  ( 0.000000000000000000, 1.000000000000000000, -0.000000000000000000 ) ) ;
#14825=VECTOR ( 'NONE', #6271, 1000.000000000000000 ) ;
#14836=ORIENTED_EDGE ( 'NONE', *, *, #4800, .F. ) ;
#14837=CARTESIAN_POINT ( 'NONE',  ( 10.18924542913430820, 0.000000000000000000, 1.000000000000000000 ) ) ;
#14849=VECTOR ( 'NONE', #7003, 1000.000000000000000 ) ;
#14852=ORIENTED_EDGE ( 'NONE', *, *, #6673, .T. ) ;
#14854=CARTESIAN_POINT ( 'NONE',  ( 5.381197846483058989, -14.00000000000000000, 2.000000000000000000 ) ) ;
#14856=DIRECTION ( 'NONE',  ( -1.000000000000000000, 0.000000000000000000, 0.000000000000000000 ) ) ;
#14857=ADVANCED_FACE ( 'NONE', ( #14931 ), #18091, .T. ) ;
#14862=CARTESIAN_POINT ( 'NONE',  ( 21.25349085826861995, 11.64110105645932691, 10.00000000000000000 ) ) ;
#14868=DIRECTION ( 'NONE',  ( 0.000000000000000000, 0.000000000000000000, -1.000000000000000000 ) ) ;
#14872=EDGE_CURVE ( 'NONE', #6318, #10660, #8362, .T. ) ;
#14887=DIRECTION ( 'NONE',  ( 1.000000000000000000, 0.000000000000000000, 0.000000000000000000 ) ) ;
#14890=DIRECTION ( 'NONE',  ( 1.000000000000000000, 0.000000000000000000, -0.000000000000000000 ) ) ;
#14896=CARTESIAN_POINT ( 'NONE',  ( -3.500698171653725765, 16.00000000000000000, 1.000000000000000000 ) ) ;
#14900=EDGE_CURVE ( 'NONE', #11113, #411, #18188, .T. ) ;
#14904=ORIENTED_EDGE ( 'NONE', *, *, #10792, .T. ) ;
#14909=LINE ( 'NONE', #5499, #5319 ) ;
#14914=CARTESIAN_POINT ( 'NONE',  ( 0.000000000000000000, 10.00000000000000000, 1.000000000000000000 ) ) ;
#14916=LINE ( 'NONE', #2260, #9625 ) ;
#14921=ORIENTED_EDGE ( 'NONE', *, *, #9122, .F. ) ;
#14925=DIRECTION ( 'NONE',  ( 3.469446951953491127E-15, 1.000000000000000000, -0.000000000000000000 ) ) ;
#14926=DIRECTION ( 'NONE',  ( 1.000000000000000000, 0.000000000000000000, -0.000000000000000000 ) ) ;
#14931=FACE_OUTER_BOUND ( 'NONE', #10639, .T. ) ;
#14935=PLANE ( 'NONE',  #11025 ) ;
#14938=CARTESIAN_POINT ( 'NONE',  ( 18.44064177244175440, 11.64110105645932691, 10.00000000000000000 ) ) ;
#14939=CARTESIAN_POINT ( 'NONE',  ( -14.56494360078803396, 11.64110105645932691, 0.000000000000000000 ) ) ;
#14944=CARTESIAN_POINT ( 'NONE',  ( 0.000000000000000000, 10.00000000000000000, 1.000000000000000000 ) ) ;
#14951=DIRECTION ( 'NONE',  ( 1.000000000000000000, 0.000000000000000000, -0.000000000000000000 ) ) ;
#14956=VECTOR ( 'NONE', #17770, 1000.000000000000000 ) ;
#14961=ADVANCED_FACE ( 'NONE', ( #16305 ), #9085, .T. ) ;
#14962=CARTESIAN_POINT ( 'NONE',  ( -26.94203811574920593, 11.64110105645932691, 0.000000000000000000 ) ) ;
#14969=EDGE_CURVE ( 'NONE', #17844, #2663, #10449, .T. ) ;
#14974=ORIENTED_EDGE ( 'NONE', *, *, #20641, .F. ) ;
#14978=DIRECTION ( 'NONE',  ( 1.000000000000000000, 0.000000000000000000, 0.000000000000000000 ) ) ;
#14979=ORIENTED_EDGE ( 'NONE', *, *, #718, .T. ) ;
#14980=ORIENTED_EDGE ( 'NONE', *, *, #5301, .F. ) ;
#14982=AXIS2_PLACEMENT_3D ( 'NONE', #16257, #5477, #11850 ) ;
#14983=CARTESIAN_POINT ( 'NONE',  ( 0.000000000000000000, 11.64110105645932691, 10.00000000000000000 ) ) ;
#14987=LINE ( 'NONE', #2031, #1984 ) ;
#14989=CARTESIAN_POINT ( 'NONE',  ( -24.12918902992234393, 11.64110105645932691, 10.00000000000000000 ) ) ;
#14996=VERTEX_POINT ( 'NONE', #12520 ) ;
#15000=VECTOR ( 'NONE', #1868, 1000.000000000000000 ) ;
#15001=ORIENTED_EDGE ( 'NONE', *, *, #2817, .T. ) ;
#15012=LINE ( 'NONE', #16577, #5990 ) ;
#15013=EDGE_CURVE ( 'NONE', #18054, #18680, #5939, .T. ) ;
#15019=VECTOR ( 'NONE', #12452, 1000.000000000000000 ) ;
#15026=ORIENTED_EDGE ( 'NONE', *, *, #17663, .F. ) ;
#15033=EDGE_LOOP ( 'NONE', ( #18961, #10151, #6098, #10823 ) ) ;
#15038=DIRECTION ( 'NONE',  ( 1.000000000000000000, 0.000000000000000000, 0.000000000000000000 ) ) ;
#15041=CARTESIAN_POINT ( 'NONE',  ( -27.94203811574921659, 9.999999999999998224, 1.000000000000000000 ) ) ;
#15047=VECTOR ( 'NONE', #16569, 1000.000000000000000 ) ;
#15049=VECTOR ( 'NONE', #11225, 1000.000000000000000 ) ;
#15050=VECTOR ( 'NONE', #3266, 1000.000000000000000 ) ;
#15053=DIRECTION ( 'NONE',  ( 0.000000000000000000, 0.000000000000000000, 1.000000000000000000 ) ) ;
#15057=CARTESIAN_POINT ( 'NONE',  ( 5.381197846483058989, -6.000000000000000000, 1.000000000000000000 ) ) ;
#15058=EDGE_LOOP ( 'NONE', ( #151, #15528, #15062, #9253 ) ) ;
#15059=ORIENTED_EDGE ( 'NONE', *, *, #13617, .F. ) ;
#15062=ORIENTED_EDGE ( 'NONE', *, *, #5535, .T. ) ;
#15071=CARTESIAN_POINT ( 'NONE',  ( -16.62779268661489951, 10.00000000000000000, 0.000000000000000000 ) ) ;
#15073=CARTESIAN_POINT ( 'NONE',  ( 30.00000000000000000, 3.000000000000000000, 1.000000000000000000 ) ) ;
#15085=VERTEX_POINT ( 'NONE', #16819 ) ;
#15086=ADVANCED_FACE ( 'NONE', ( #13779 ), #4480, .T. ) ;
#15089=DIRECTION ( 'NONE',  ( 0.000000000000000000, 0.000000000000000000, 1.000000000000000000 ) ) ;
#15090=DIRECTION ( 'NONE',  ( 0.000000000000000000, 1.000000000000000000, -0.000000000000000000 ) ) ;
#15091=EDGE_CURVE ( 'NONE', #15857, #8796, #16324, .T. ) ;
#15092=EDGE_CURVE ( 'NONE', #5162, #12182, #15659, .T. ) ;
#15093=CARTESIAN_POINT ( 'NONE',  ( 5.381197846483058989, -14.00000000000000000, 2.000000000000000000 ) ) ;
#15104=ORIENTED_EDGE ( 'NONE', *, *, #5687, .F. ) ;
#15113=VERTEX_POINT ( 'NONE', #17021 ) ;
#15117=EDGE_CURVE ( 'NONE', #12575, #14721, #13879, .T. ) ;
#15120=EDGE_CURVE ( 'NONE', #5545, #20631, #6980, .T. ) ;
#15125=DIRECTION ( 'NONE',  ( 1.000000000000000000, 0.000000000000000000, 0.000000000000000000 ) ) ;
#15136=ORIENTED_EDGE ( 'NONE', *, *, #12931, .F. ) ;
#15141=EDGE_CURVE ( 'NONE', #6665, #19457, #20495, .T. ) ;
#15142=CARTESIAN_POINT ( 'NONE',  ( 7.500000000000002665, -9.999999999999991118, 2.000000000000000000 ) ) ;
#15143=ORIENTED_EDGE ( 'NONE', *, *, #19705, .F. ) ;
#15147=DIRECTION ( 'NONE',  ( -0.000000000000000000, -0.000000000000000000, -1.000000000000000000 ) ) ;
#15177=DIRECTION ( 'NONE',  ( -0.000000000000000000, 0.000000000000000000, -1.000000000000000000 ) ) ;
#15182=CARTESIAN_POINT ( 'NONE',  ( 0.000000000000000000, 16.00000000000000000, 1.000000000000000000 ) ) ;
#15194=AXIS2_PLACEMENT_3D ( 'NONE', #12034, #18428, #16846 ) ;
#15197=CARTESIAN_POINT ( 'NONE',  ( 27.00000000000000000, 3.000000000000000000, 0.000000000000000000 ) ) ;
#15199=CARTESIAN_POINT ( 'NONE',  ( -15.87779268661489773, 10.00000000000000000, 1.000000000000000000 ) ) ;
#15201=EDGE_CURVE ( 'NONE', #17667, #7935, #14909, .T. ) ;
#15202=CARTESIAN_POINT ( 'NONE',  ( 10.38119784648305810, -14.00000000000000000, 2.000000000000000000 ) ) ;
#15205=ORIENTED_EDGE ( 'NONE', *, *, #17827, .T. ) ;
#15210=ORIENTED_EDGE ( 'NONE', *, *, #20235, .T. ) ;
#15212=LINE ( 'NONE', #7273, #3368 ) ;
#15221=CARTESIAN_POINT ( 'NONE',  ( -24.12918902992234393, 10.00000000000000000, 1.000000000000000000 ) ) ;
#15229=PLANE ( 'NONE',  #14340 ) ;
#15238=EDGE_LOOP ( 'NONE', ( #8329, #14407, #15001, #14389 ) ) ;
#15242=EDGE_LOOP ( 'NONE', ( #5522, #7018, #16208, #5713 ) ) ;
#15245=DIRECTION ( 'NONE',  ( -0.000000000000000000, 0.000000000000000000, -1.000000000000000000 ) ) ;
#15246=LINE ( 'NONE', #10341, #14639 ) ;
#15260=CARTESIAN_POINT ( 'NONE',  ( -7.626396343307448866, 11.64110105645932691, 0.000000000000000000 ) ) ;
#15261=ORIENTED_EDGE ( 'NONE', *, *, #9150, .T. ) ;
#15262=VERTEX_POINT ( 'NONE', #13037 ) ;
#15266=PLANE ( 'NONE',  #9789 ) ;
#15267=DIRECTION ( 'NONE',  ( 0.000000000000000000, -0.000000000000000000, 1.000000000000000000 ) ) ;
#15269=DIRECTION ( 'NONE',  ( 5.782411586589356653E-16, -1.000000000000000000, 0.000000000000000000 ) ) ;
#15273=EDGE_CURVE ( 'NONE', #886, #14781, #3620, .T. ) ;
#15279=EDGE_CURVE ( 'NONE', #4668, #6506, #4242, .T. ) ;
#15284=ORIENTED_EDGE ( 'NONE', *, *, #17331, .F. ) ;
#15287=ORIENTED_EDGE ( 'NONE', *, *, #11261, .T. ) ;
#15289=ADVANCED_FACE ( 'NONE', ( #7181 ), #15431, .T. ) ;
#15296=CARTESIAN_POINT ( 'NONE',  ( -7.626396343307448866, 11.64110105645932691, 10.00000000000000000 ) ) ;
#15298=DIRECTION ( 'NONE',  ( -1.000000000000000000, 0.000000000000000000, 0.000000000000000000 ) ) ;
#15301=DIRECTION ( 'NONE',  ( 1.000000000000000000, -0.000000000000000000, -0.000000000000000000 ) ) ;
#15304=VERTEX_POINT ( 'NONE', #12187 ) ;
#15306=CARTESIAN_POINT ( 'NONE',  ( -7.626396343307448866, 16.00000000000000000, 1.000000000000000000 ) ) ;
#15313=VERTEX_POINT ( 'NONE', #5604 ) ;
#15316=VECTOR ( 'NONE', #14010, 1000.000000000000000 ) ;
#15319=ORIENTED_EDGE ( 'NONE', *, *, #690, .T. ) ;
#15322=AXIS2_PLACEMENT_3D ( 'NONE', #9286, #20500, #4578 ) ;
#15323=LINE ( 'NONE', #1003, #10994 ) ;
#15324=AXIS2_PLACEMENT_3D ( 'NONE', #19949, #7184, #15125 ) ;
#15333=DIRECTION ( 'NONE',  ( 0.000000000000000000, -1.000000000000000000, 0.000000000000000000 ) ) ;
#15342=EDGE_LOOP ( 'NONE', ( #16481, #18419, #15261, #5753 ) ) ;
#15347=AXIS2_PLACEMENT_3D ( 'NONE', #5738, #14926, #10542 ) ;
#15349=CARTESIAN_POINT ( 'NONE',  ( 0.000000000000000000, 10.00000000000000000, 1.000000000000000000 ) ) ;
#15361=VERTEX_POINT ( 'NONE', #17104 ) ;
#15363=LINE ( 'NONE', #8791, #10751 ) ;
#15368=EDGE_LOOP ( 'NONE', ( #11678, #19318, #7892, #9159 ) ) ;
#15371=DIRECTION ( 'NONE',  ( -0.000000000000000000, -0.000000000000000000, -1.000000000000000000 ) ) ;
#15384=LINE ( 'NONE', #2837, #11066 ) ;
#15392=EDGE_LOOP ( 'NONE', ( #5214, #17324, #13274, #10472 ) ) ;
#15394=LINE ( 'NONE', #4003, #10350 ) ;
#15396=ADVANCED_FACE ( 'NONE', ( #20052 ), #9060, .T. ) ;
#15397=VECTOR ( 'NONE', #20132, 1000.000000000000114 ) ;
#15405=CARTESIAN_POINT ( 'NONE',  ( -0.000000000000000000, 10.00000000000000000, 0.000000000000000000 ) ) ;
#15407=DIRECTION ( 'NONE',  ( 0.000000000000000000, -0.000000000000000000, 1.000000000000000000 ) ) ;
#15408=ADVANCED_FACE ( 'NONE', ( #7590 ), #12087, .F. ) ;
#15421=EDGE_LOOP ( 'NONE', ( #14974, #7356, #172, #4671 ) ) ;
#15431=CYLINDRICAL_SURFACE ( 'NONE', #9000, 10.00000000000000000 ) ;
#15438=ADVANCED_FACE ( 'NONE', ( #15629 ), #13545, .T. ) ;
#15443=CYLINDRICAL_SURFACE ( 'NONE', #3542, 10.00000000000000000 ) ;
#15451=ORIENTED_EDGE ( 'NONE', *, *, #19919, .F. ) ;
#15453=ORIENTED_EDGE ( 'NONE', *, *, #2460, .T. ) ;
#15458=CARTESIAN_POINT ( 'NONE',  ( -26.94203811574920593, 10.00000000000000000, 1.000000000000000000 ) ) ;
#15472=CARTESIAN_POINT ( 'NONE',  ( 14.31494360078803041, 0.000000000000000000, 0.000000000000000000 ) ) ;
#15476=DIRECTION ( 'NONE',  ( 1.000000000000000000, 0.000000000000000000, 0.000000000000000000 ) ) ;
#15477=ORIENTED_EDGE ( 'NONE', *, *, #1314, .T. ) ;
#15481=CARTESIAN_POINT ( 'NONE',  ( 26.69203811574920948, 1.543443504701929706E-14, 1.000000000000000000 ) ) ;
#15488=EDGE_CURVE ( 'NONE', #18502, #17840, #13090, .T. ) ;
#15494=EDGE_CURVE ( 'NONE', #19407, #15727, #19385, .T. ) ;
#15498=ORIENTED_EDGE ( 'NONE', *, *, #10836, .F. ) ;
#15501=DIRECTION ( 'NONE',  ( 1.000000000000000000, 0.000000000000000000, 0.000000000000000000 ) ) ;
#15507=CARTESIAN_POINT ( 'NONE',  ( -15.00000000000000000, 3.000000000000000000, 1.000000000000000000 ) ) ;
#15508=CARTESIAN_POINT ( 'NONE',  ( 0.000000000000000000, 10.00000000000000000, 1.000000000000000000 ) ) ;
#15509=EDGE_CURVE ( 'NONE', #7326, #6555, #14656, .T. ) ;
#15510=CARTESIAN_POINT ( 'NONE',  ( -24.12918902992234393, 0.000000000000000000, 1.000000000000000000 ) ) ;
#15513=ORIENTED_EDGE ( 'NONE', *, *, #8097, .T. ) ;
#15515=PLANE ( 'NONE',  #7046 ) ;
#15521=VERTEX_POINT ( 'NONE', #7801 ) ;
#15522=ORIENTED_EDGE ( 'NONE', *, *, #13573, .T. ) ;
#15523=DIRECTION ( 'NONE',  ( 1.000000000000000000, -0.000000000000000000, 0.000000000000000000 ) ) ;
#15524=EDGE_LOOP ( 'NONE', ( #16881, #10616, #6887, #2637 ) ) ;
#15528=ORIENTED_EDGE ( 'NONE', *, *, #13257, .F. ) ;
#15529=DIRECTION ( 'NONE',  ( 0.000000000000000000, 0.000000000000000000, -1.000000000000000000 ) ) ;
#15535=CARTESIAN_POINT ( 'NONE',  ( -8.376396343307449754, 10.00000000000000000, 0.000000000000000000 ) ) ;
#15540=EDGE_CURVE ( 'NONE', #20714, #13339, #2007, .T. ) ;
#15548=ORIENTED_EDGE ( 'NONE', *, *, #11713, .F. ) ;
#15555=EDGE_CURVE ( 'NONE', #1608, #12080, #17805, .T. ) ;
#15558=DIRECTION ( 'NONE',  ( 1.000000000000000000, -0.000000000000000000, 0.000000000000000000 ) ) ;
#15564=DIRECTION ( 'NONE',  ( 0.000000000000000000, 1.000000000000000000, 0.000000000000000000 ) ) ;
#15566=ORIENTED_EDGE ( 'NONE', *, *, #8470, .T. ) ;
#15568=LINE ( 'NONE', #7119, #14758 ) ;
#15572=ORIENTED_EDGE ( 'NONE', *, *, #17457, .F. ) ;
#15576=ORIENTED_EDGE ( 'NONE', *, *, #18885, .T. ) ;
#15592=ORIENTED_EDGE ( 'NONE', *, *, #7235, .T. ) ;
#15607=EDGE_CURVE ( 'NONE', #682, #3633, #5241, .T. ) ;
#15614=CARTESIAN_POINT ( 'NONE',  ( -26.19203811574920593, 0.000000000000000000, 1.000000000000000000 ) ) ;
#15621=ORIENTED_EDGE ( 'NONE', *, *, #9559, .T. ) ;
#15623=EDGE_LOOP ( 'NONE', ( #14921, #9149, #17584, #2668 ) ) ;
#15625=EDGE_CURVE ( 'NONE', #16502, #351, #18006, .T. ) ;
#15629=FACE_OUTER_BOUND ( 'NONE', #15524, .T. ) ;
#15648=CARTESIAN_POINT ( 'NONE',  ( 9.000000000000000000, -9.999999999999991118, 1.000000000000000000 ) ) ;
#15651=DIRECTION ( 'NONE',  ( 0.000000000000000000, -1.000000000000000000, 0.000000000000000000 ) ) ;
#15656=VECTOR ( 'NONE', #5403, 1000.000000000000000 ) ;
#15659=LINE ( 'NONE', #18709, #15991 ) ;
#15660=CARTESIAN_POINT ( 'NONE',  ( 0.000000000000000000, 10.00000000000000000, 1.000000000000000000 ) ) ;
#15666=PLANE ( 'NONE',  #5524 ) ;
#15671=LINE ( 'NONE', #6370, #2392 ) ;
#15673=AXIS2_PLACEMENT_3D ( 'NONE', #2786, #17305, #9162 ) ;
#15674=VECTOR ( 'NONE', #7182, 1000.000000000000000 ) ;
#15678=ORIENTED_EDGE ( 'NONE', *, *, #14394, .T. ) ;
#15682=ORIENTED_EDGE ( 'NONE', *, *, #18479, .T. ) ;
#15684=EDGE_CURVE ( 'NONE', #4496, #351, #11865, .T. ) ;
#15690=CIRCLE ( 'NONE', #8004, 10.00000000000000000 ) ;
#15691=CARTESIAN_POINT ( 'NONE',  ( -2.187849085826861550, 10.00000000000000000, 1.000000000000000000 ) ) ;
#15705=VERTEX_POINT ( 'NONE', #19800 ) ;
#15712=DIRECTION ( 'NONE',  ( 0.1736481776669292765, -0.9848077530122082424, 0.000000000000000000 ) ) ;
#15727=VERTEX_POINT ( 'NONE', #8697 ) ;
#15728=VECTOR ( 'NONE', #13704, 1000.000000000000000 ) ;
#15730=DIRECTION ( 'NONE',  ( -0.000000000000000000, -0.000000000000000000, -1.000000000000000000 ) ) ;
#15732=ORIENTED_EDGE ( 'NONE', *, *, #2066, .T. ) ;
#15733=ORIENTED_EDGE ( 'NONE', *, *, #11710, .F. ) ;
#15742=CARTESIAN_POINT ( 'NONE',  ( 15.06494360078803041, 11.64110105645932691, 10.00000000000000000 ) ) ;
#15743=CARTESIAN_POINT ( 'NONE',  ( -4.250698171653726654, 10.00000000000000000, 0.000000000000000000 ) ) ;
#15750=EDGE_CURVE ( 'NONE', #7608, #11568, #10163, .T. ) ;
#15754=DIRECTION ( 'NONE',  ( -1.000000000000000000, 0.000000000000000000, 0.000000000000000000 ) ) ;
#15758=ORIENTED_EDGE ( 'NONE', *, *, #9122, .T. ) ;
#15771=LINE ( 'NONE', #17546, #16221 ) ;
#15778=ORIENTED_EDGE ( 'NONE', *, *, #8695, .F. ) ;
#15779=AXIS2_PLACEMENT_3D ( 'NONE', #2979, #12973, #14442 ) ;
#15781=LINE ( 'NONE', #7433, #20367 ) ;
#15782=ORIENTED_EDGE ( 'NONE', *, *, #3778, .F. ) ;
#15783=CARTESIAN_POINT ( 'NONE',  ( -0.000000000000000000, 11.64110105645932691, 0.000000000000000000 ) ) ;
#15787=DIRECTION ( 'NONE',  ( 1.000000000000000000, 1.734723475976787570E-15, 0.000000000000000000 ) ) ;
#15793=DIRECTION ( 'NONE',  ( 1.000000000000000000, 0.000000000000000000, 0.000000000000000000 ) ) ;
#15814=DIRECTION ( 'NONE',  ( 1.000000000000000000, 0.000000000000000000, 0.000000000000000000 ) ) ;
#15815=DIRECTION ( 'NONE',  ( 0.000000000000000000, 0.000000000000000000, -1.000000000000000000 ) ) ;
#15816=CARTESIAN_POINT ( 'NONE',  ( 4.750698171653723989, 0.000000000000000000, 1.000000000000000000 ) ) ;
#15822=AXIS2_PLACEMENT_3D ( 'NONE', #20524, #6177, #7444 ) ;
#15823=VERTEX_POINT ( 'NONE', #850 ) ;
#15825=CARTESIAN_POINT ( 'NONE',  ( 0.000000000000000000, 0.000000000000000000, 1.000000000000000000 ) ) ;
#15828=EDGE_LOOP ( 'NONE', ( #7895, #4955, #12231, #576 ) ) ;
#15835=ADVANCED_FACE ( 'NONE', ( #7232 ), #19998, .T. ) ;
#15836=DIRECTION ( 'NONE',  ( 0.000000000000000000, 1.000000000000000000, -0.000000000000000000 ) ) ;
#15843=DIRECTION ( 'NONE',  ( 1.000000000000000000, 0.000000000000000000, 0.000000000000000000 ) ) ;
#15845=CARTESIAN_POINT ( 'NONE',  ( 10.49999999999999467, -9.999999999999991118, 2.000000000000000000 ) ) ;
#15852=ORIENTED_EDGE ( 'NONE', *, *, #4137, .F. ) ;
#15854=CARTESIAN_POINT ( 'NONE',  ( -22.81633994409548549, 11.64110105645932691, 10.00000000000000000 ) ) ;
#15855=EDGE_LOOP ( 'NONE', ( #17716, #3487, #14692, #13796 ) ) ;
#15856=LINE ( 'NONE', #1535, #18679 ) ;
#15857=VERTEX_POINT ( 'NONE', #5769 ) ;
#15864=VECTOR ( 'NONE', #8283, 1000.000000000000000 ) ;
#15873=VECTOR ( 'NONE', #8114, 1000.000000000000000 ) ;
#15907=CIRCLE ( 'NONE', #6897, 10.00000000000000000 ) ;
#15908=CARTESIAN_POINT ( 'NONE',  ( -2.187849085826861550, 0.000000000000000000, 1.000000000000000000 ) ) ;
#15913=CYLINDRICAL_SURFACE ( 'NONE', #16359, 10.00000000000000000 ) ;
#15923=LINE ( 'NONE', #3274, #11380 ) ;
#15932=VERTEX_POINT ( 'NONE', #10890 ) ;
#15934=CARTESIAN_POINT ( 'NONE',  ( -24.12918902992234393, 0.000000000000000000, 0.000000000000000000 ) ) ;
#15941=DIRECTION ( 'NONE',  ( -0.000000000000000000, -0.000000000000000000, -1.000000000000000000 ) ) ;
#15943=CARTESIAN_POINT ( 'NONE',  ( 27.94203811574921659, 9.999999999999998224, 1.000000000000000000 ) ) ;
#15944=CARTESIAN_POINT ( 'NONE',  ( -3.500698171653725765, 10.00000000000000000, 0.000000000000000000 ) ) ;
#15953=DIRECTION ( 'NONE',  ( 0.000000000000000000, 0.000000000000000000, -1.000000000000000000 ) ) ;
#15958=DIRECTION ( 'NONE',  ( 0.000000000000000000, 1.000000000000000000, 0.000000000000000000 ) ) ;
#15961=PRODUCT_DEFINITION ( 'UNKNOWN', '', #7040, #4614 ) ;
#15964=DIRECTION ( 'NONE',  ( -0.000000000000000000, -0.000000000000000000, -1.000000000000000000 ) ) ;
#15966=CARTESIAN_POINT ( 'NONE',  ( -30.00000000000000000, 0.000000000000000000, 1.000000000000000000 ) ) ;
#15969=LINE ( 'NONE', #9806, #13970 ) ;
#15971=VECTOR ( 'NONE', #11370, 1000.000000000000000 ) ;
#15984=LINE ( 'NONE', #15783, #19966 ) ;
#15987=VECTOR ( 'NONE', #12599, 1000.000000000000000 ) ;
#15991=VECTOR ( 'NONE', #12113, 1000.000000000000000 ) ;
#15994=LINE ( 'NONE', #1468, #16279 ) ;
#15999=AXIS2_PLACEMENT_3D ( 'NONE', #18142, #665, #7054 ) ;
#16007=VECTOR ( 'NONE', #4456, 1000.000000000000000 ) ;
#16008=ADVANCED_FACE ( 'NONE', ( #14117 ), #9113, .T. ) ;
#16011=ORIENTED_EDGE ( 'NONE', *, *, #9408, .T. ) ;
#16012=ORIENTED_EDGE ( 'NONE', *, *, #5913, .T. ) ;
#16014=CARTESIAN_POINT ( 'NONE',  ( 2.687849085826861995, 10.00000000000000000, 0.000000000000000000 ) ) ;
#16015=DIRECTION ( 'NONE',  ( 0.000000000000000000, 0.000000000000000000, 1.000000000000000000 ) ) ;
#16016=ORIENTED_EDGE ( 'NONE', *, *, #20383, .F. ) ;
#16019=EDGE_CURVE ( 'NONE', #9844, #12110, #13806, .T. ) ;
#16026=DIRECTION ( 'NONE',  ( -0.000000000000000000, 0.000000000000000000, -1.000000000000000000 ) ) ;
#16035=AXIS2_PLACEMENT_3D ( 'NONE', #7998, #20360, #9468 ) ;
#16037=DIRECTION ( 'NONE',  ( -0.1736481776669293042, 0.9848077530122082424, 0.000000000000000000 ) ) ;
#16042=EDGE_LOOP ( 'NONE', ( #2175, #793, #13632, #4895 ) ) ;
#16046=CARTESIAN_POINT ( 'NONE',  ( 1.937849085826861328, 11.64110105645932691, 0.000000000000000000 ) ) ;
#16050=LINE ( 'NONE', #19302, #11768 ) ;
#16060=VECTOR ( 'NONE', #4126, 1000.000000000000000 ) ;
#16073=DIRECTION ( 'NONE',  ( -0.000000000000000000, -0.000000000000000000, -1.000000000000000000 ) ) ;
#16075=ORIENTED_EDGE ( 'NONE', *, *, #7869, .T. ) ;
#16078=PLANE ( 'NONE',  #19809 ) ;
#16080=VECTOR ( 'NONE', #3883, 1000.000000000000000 ) ;
#16088=CARTESIAN_POINT ( 'NONE',  ( 2.687849085826861995, 0.000000000000000000, 1.000000000000000000 ) ) ;
#16090=CARTESIAN_POINT ( 'NONE',  ( 23.31633994409548549, 0.000000000000000000, 0.000000000000000000 ) ) ;
#16093=VERTEX_POINT ( 'NONE', #17671 ) ;
#16102=VERTEX_POINT ( 'NONE', #11191 ) ;
#16103=LINE ( 'NONE', #7747, #16472 ) ;
#16104=EDGE_LOOP ( 'NONE', ( #14701, #17655, #10832, #18390, #15782, #3362 ) ) ;
#16106=CIRCLE ( 'NONE', #13767, 1.499999999999996225 ) ;
#16107=LINE ( 'NONE', #1672, #14256 ) ;
#16110=ADVANCED_FACE ( 'NONE', ( #1567 ), #1878, .F. ) ;
#16122=ORIENTED_EDGE ( 'NONE', *, *, #19410, .F. ) ;
#16123=ORIENTED_EDGE ( 'NONE', *, *, #6668, .F. ) ;
#16125=CARTESIAN_POINT ( 'NONE',  ( -24.87918902992234393, 0.000000000000000000, 0.000000000000000000 ) ) ;
#16126=LINE ( 'NONE', #5032, #6024 ) ;
#16128=ORIENTED_EDGE ( 'NONE', *, *, #12166, .F. ) ;
#16134=CARTESIAN_POINT ( 'NONE',  ( 0.000000000000000000, 10.00000000000000000, 1.000000000000000000 ) ) ;
#16140=PLANE ( 'NONE',  #2729 ) ;
#16143=EDGE_CURVE ( 'NONE', #7302, #11608, #19358, .T. ) ;
#16149=VECTOR ( 'NONE', #2391, 1000.000000000000000 ) ;
#16154=DIRECTION ( 'NONE',  ( 1.000000000000000000, 0.000000000000000000, -0.000000000000000000 ) ) ;
#16159=DIRECTION ( 'NONE',  ( 0.000000000000000000, -1.000000000000000000, 0.000000000000000000 ) ) ;
#16166=CARTESIAN_POINT ( 'NONE',  ( 10.49999999999999645, -9.999999999999991118, 2.000000000000000000 ) ) ;
#16172=ORIENTED_EDGE ( 'NONE', *, *, #18812, .T. ) ;
#16183=DIRECTION ( 'NONE',  ( 1.000000000000000000, 0.000000000000000000, 0.000000000000000000 ) ) ;
#16186=LINE ( 'NONE', #1853, #1322 ) ;
#16190=LINE ( 'NONE', #9699, #20707 ) ;
#16193=FILL_AREA_STYLE_COLOUR ( '', #16968 ) ;
#16197=VERTEX_POINT ( 'NONE', #309 ) ;
#16202=EDGE_CURVE ( 'NONE', #12110, #7216, #6695, .T. ) ;
#16206=ORIENTED_EDGE ( 'NONE', *, *, #3114, .F. ) ;
#16208=ORIENTED_EDGE ( 'NONE', *, *, #13497, .F. ) ;
#16212=AXIS2_PLACEMENT_3D ( 'NONE', #15742, #4859, #6329 ) ;
#16220=LINE ( 'NONE', #8269, #19122 ) ;
#16221=VECTOR ( 'NONE', #8038, 1000.000000000000000 ) ;
#16226=EDGE_LOOP ( 'NONE', ( #4389, #13007, #8825, #6832 ) ) ;
#16228=DIRECTION ( 'NONE',  ( -1.000000000000000000, 0.000000000000000000, 0.000000000000000000 ) ) ;
#16229=DIRECTION ( 'NONE',  ( 0.000000000000000000, 0.000000000000000000, 1.000000000000000000 ) ) ;
#16232=DIRECTION ( 'NONE',  ( 0.000000000000000000, 0.000000000000000000, 1.000000000000000000 ) ) ;
#16236=CARTESIAN_POINT ( 'NONE',  ( -0.000000000000000000, 10.00000000000000000, 0.000000000000000000 ) ) ;
#16239=DIRECTION ( 'NONE',  ( 1.000000000000000000, 0.000000000000000000, -0.000000000000000000 ) ) ;
#16244=DIRECTION ( 'NONE',  ( 1.000000000000000000, 0.000000000000000000, 0.000000000000000000 ) ) ;
#16247=VERTEX_POINT ( 'NONE', #7311 ) ;
#16251=ORIENTED_EDGE ( 'NONE', *, *, #18029, .F. ) ;
#16252=EDGE_CURVE ( 'NONE', #10437, #4996, #10236, .T. ) ;
#16257=CARTESIAN_POINT ( 'NONE',  ( 0.000000000000000000, 11.64110105645932691, 10.00000000000000000 ) ) ;
#16266=EDGE_LOOP ( 'NONE', ( #3229, #20555, #5088, #14388 ) ) ;
#16276=EDGE_CURVE ( 'NONE', #10193, #3754, #6893, .T. ) ;
#16278=DIRECTION ( 'NONE',  ( 0.000000000000000000, -0.000000000000000000, 1.000000000000000000 ) ) ;
#16279=VECTOR ( 'NONE', #17466, 1000.000000000000000 ) ;
#16282=CARTESIAN_POINT ( 'NONE',  ( -4.250698171653726654, 11.64110105645932691, 10.00000000000000000 ) ) ;
#16287=( LENGTH_UNIT ( ) NAMED_UNIT ( * ) SI_UNIT ( .MILLI., .METRE. ) );
#16296=DIRECTION ( 'NONE',  ( -1.000000000000000000, 3.469446951953491127E-15, 0.000000000000000000 ) ) ;
#16297=EDGE_CURVE ( 'NONE', #13178, #13945, #17980, .T. ) ;
#16303=FACE_OUTER_BOUND ( 'NONE', #16792, .T. ) ;
#16305=FACE_OUTER_BOUND ( 'NONE', #10418, .T. ) ;
#16308=EDGE_CURVE ( 'NONE', #9894, #11041, #13263, .T. ) ;
#16316=LINE ( 'NONE', #3457, #18114 ) ;
#16319=AXIS2_PLACEMENT_3D ( 'NONE', #16843, #19996, #748 ) ;
#16321=ADVANCED_FACE ( 'NONE', ( #19974 ), #16511, .T. ) ;
#16324=CIRCLE ( 'NONE', #7653, 1.499999999999998668 ) ;
#16326=PRESENTATION_STYLE_ASSIGNMENT (( #9944 ) ) ;
#16335=VECTOR ( 'NONE', #14730, 1000.000000000000000 ) ;
#16339=CARTESIAN_POINT ( 'NONE',  ( -13.81494360078803396, 10.00000000000000000, 1.000000000000000000 ) ) ;
#16342=FACE_OUTER_BOUND ( 'NONE', #1130, .T. ) ;
#16348=VECTOR ( 'NONE', #11644, 1000.000000000000000 ) ;
#16353=CARTESIAN_POINT ( 'NONE',  ( 26.69203811574920238, 10.00000000000000000, 1.000000000000000000 ) ) ;
#16354=CARTESIAN_POINT ( 'NONE',  ( -0.000000000000000000, 11.64110105645932691, 0.000000000000000000 ) ) ;
#16359=AXIS2_PLACEMENT_3D ( 'NONE', #226, #1801, #1590 ) ;
#16363=CARTESIAN_POINT ( 'NONE',  ( -15.87779268661489773, 0.000000000000000000, 1.000000000000000000 ) ) ;
#16369=CIRCLE ( 'NONE', #6360, 10.00000000000000000 ) ;
#16380=EDGE_LOOP ( 'NONE', ( #11389, #17047, #13890, #18470 ) ) ;
#16387=EDGE_CURVE ( 'NONE', #12514, #10855, #13571, .T. ) ;
#16393=EDGE_LOOP ( 'NONE', ( #1840, #7318, #6836, #11137 ) ) ;
#16404=EDGE_LOOP ( 'NONE', ( #7542, #4135, #11270, #7072 ) ) ;
#16412=EDGE_CURVE ( 'NONE', #13481, #13250, #616, .T. ) ;
#16418=CARTESIAN_POINT ( 'NONE',  ( 0.000000000000000000, 0.000000000000000000, 0.000000000000000000 ) ) ;
#16419=DIRECTION ( 'NONE',  ( 1.000000000000000000, 0.000000000000000000, -0.000000000000000000 ) ) ;
#16426=( NAMED_UNIT ( * ) PLANE_ANGLE_UNIT ( ) SI_UNIT ( $, .RADIAN. ) );
#16427=EDGE_LOOP ( 'NONE', ( #19652, #20041, #19345, #14643 ) ) ;
#16428=EDGE_CURVE ( 'NONE', #13538, #12998, #2282, .T. ) ;
#16438=CARTESIAN_POINT ( 'NONE',  ( 10.18924542913430820, 0.000000000000000000, 0.000000000000000000 ) ) ;
#16441=CARTESIAN_POINT ( 'NONE',  ( -0.000000000000000000, 10.00000000000000000, 0.000000000000000000 ) ) ;
#16453=ORIENTED_EDGE ( 'NONE', *, *, #11065, .F. ) ;
#16456=LINE ( 'NONE', #11947, #19150 ) ;
#16458=CARTESIAN_POINT ( 'NONE',  ( -16.62779268661489951, 0.000000000000000000, 1.000000000000000000 ) ) ;
#16459=FACE_OUTER_BOUND ( 'NONE', #1970, .T. ) ;
#16464=AXIS2_PLACEMENT_3D ( 'NONE', #18293, #18405, #3858 ) ;
#16465=CARTESIAN_POINT ( 'NONE',  ( 0.000000000000000000, 16.00000000000000000, 1.000000000000000000 ) ) ;
#16472=VECTOR ( 'NONE', #19152, 1000.000000000000000 ) ;
#16476=DIRECTION ( 'NONE',  ( 1.000000000000000000, 0.000000000000000000, 0.000000000000000000 ) ) ;
#16478=ORIENTED_EDGE ( 'NONE', *, *, #16019, .T. ) ;
#16480=DIRECTION ( 'NONE',  ( 0.000000000000000000, -1.000000000000000000, 0.000000000000000000 ) ) ;
#16481=ORIENTED_EDGE ( 'NONE', *, *, #9559, .F. ) ;
#16482=DIRECTION ( 'NONE',  ( 1.000000000000000000, 0.000000000000000000, 0.000000000000000000 ) ) ;
#16483=EDGE_LOOP ( 'NONE', ( #2153, #5841, #1306, #18080 ) ) ;
#16499=PLANE ( 'NONE',  #5622 ) ;
#16502=VERTEX_POINT ( 'NONE', #12317 ) ;
#16505=ORIENTED_EDGE ( 'NONE', *, *, #3355, .T. ) ;
#16506=DIRECTION ( 'NONE',  ( 0.000000000000000000, 0.000000000000000000, 1.000000000000000000 ) ) ;
#16510=DIRECTION ( 'NONE',  ( 1.000000000000000000, 0.000000000000000000, -0.000000000000000000 ) ) ;
#16511=PLANE ( 'NONE',  #16464 ) ;
#16518=FACE_OUTER_BOUND ( 'NONE', #6119, .T. ) ;
#16519=CARTESIAN_POINT ( 'NONE',  ( 13.00209451496117374, 0.000000000000000000, 1.000000000000000000 ) ) ;
#16525=DIRECTION ( 'NONE',  ( 0.000000000000000000, -0.000000000000000000, 1.000000000000000000 ) ) ;
#16528=DIRECTION ( 'NONE',  ( 0.000000000000000000, 0.000000000000000000, 1.000000000000000000 ) ) ;
#16540=DIRECTION ( 'NONE',  ( 0.000000000000000000, 0.000000000000000000, 1.000000000000000000 ) ) ;
#16547=DIRECTION ( 'NONE',  ( -1.000000000000000000, 0.000000000000000000, 0.000000000000000000 ) ) ;
#16550=ORIENTED_EDGE ( 'NONE', *, *, #20048, .T. ) ;
#16553=CARTESIAN_POINT ( 'NONE',  ( 10.93924542913430820, 10.00000000000000000, 0.000000000000000000 ) ) ;
#16560=CARTESIAN_POINT ( 'NONE',  ( -22.06633994409548194, 0.000000000000000000, 1.000000000000000000 ) ) ;
#16569=DIRECTION ( 'NONE',  ( 1.000000000000000000, 0.000000000000000000, 0.000000000000000000 ) ) ;
#16572=LINE ( 'NONE', #2249, #696 ) ;
#16573=ORIENTED_EDGE ( 'NONE', *, *, #4910, .T. ) ;
#16577=CARTESIAN_POINT ( 'NONE',  ( 27.44203811574919882, 0.000000000000000000, 1.000000000000000000 ) ) ;
#16588=ORIENTED_EDGE ( 'NONE', *, *, #13121, .F. ) ;
#16592=CARTESIAN_POINT ( 'NONE',  ( -6.313547257480587760, 0.000000000000000000, 1.000000000000000000 ) ) ;
#16598=CARTESIAN_POINT ( 'NONE',  ( -0.000000000000000000, 10.00000000000000000, 0.000000000000000000 ) ) ;
#16601=CARTESIAN_POINT ( 'NONE',  ( -24.87918902992234393, 0.000000000000000000, 1.000000000000000000 ) ) ;
#16608=EDGE_CURVE ( 'NONE', #8195, #6243, #13985, .T. ) ;
#16619=EDGE_CURVE ( 'NONE', #18960, #5420, #1143, .T. ) ;
#16621=( NAMED_UNIT ( * ) SI_UNIT ( $, .STERADIAN. ) SOLID_ANGLE_UNIT ( ) );
#16622=ORIENTED_EDGE ( 'NONE', *, *, #18885, .F. ) ;
#16637=FACE_OUTER_BOUND ( 'NONE', #16380, .T. ) ;
#16641=ORIENTED_EDGE ( 'NONE', *, *, #9359, .F. ) ;
#16645=EDGE_CURVE ( 'NONE', #15085, #7740, #4268, .T. ) ;
#16646=CARTESIAN_POINT ( 'NONE',  ( 0.000000000000000000, 11.64110105645932691, 10.00000000000000000 ) ) ;
#16651=DIRECTION ( 'NONE',  ( 0.000000000000000000, 1.000000000000000000, -0.000000000000000000 ) ) ;
#16652=AXIS2_PLACEMENT_3D ( 'NONE', #5380, #14890, #8622 ) ;
#16665=ORIENTED_EDGE ( 'NONE', *, *, #2817, .F. ) ;
#16666=VECTOR ( 'NONE', #1754, 1000.000000000000000 ) ;
#16674=DIRECTION ( 'NONE',  ( -0.000000000000000000, -0.000000000000000000, -1.000000000000000000 ) ) ;
#16680=VECTOR ( 'NONE', #10622, 1000.000000000000000 ) ;
#16684=AXIS2_PLACEMENT_3D ( 'NONE', #9630, #17481, #11208 ) ;
#16692=EDGE_CURVE ( 'NONE', #16247, #3875, #17644, .T. ) ;
#16700=CIRCLE ( 'NONE', #17708, 10.00000000000000000 ) ;
#16701=EDGE_LOOP ( 'NONE', ( #20409, #19327, #1466, #11007 ) ) ;
#16710=DIRECTION ( 'NONE',  ( 1.000000000000000000, -1.156482317317871133E-15, 0.000000000000000000 ) ) ;
#16717=LINE ( 'NONE', #5749, #1007 ) ;
#16724=VECTOR ( 'NONE', #7236, 1000.000000000000000 ) ;
#16727=LINE ( 'NONE', #17037, #11414 ) ;
#16729=VECTOR ( 'NONE', #3597, 1000.000000000000000 ) ;
#16732=EDGE_LOOP ( 'NONE', ( #20281, #16251, #10747, #19532 ) ) ;
#16736=EDGE_LOOP ( 'NONE', ( #3848, #17193, #10700, #18368 ) ) ;
#16740=AXIS2_PLACEMENT_3D ( 'NONE', #16772, #9037, #14041 ) ;
#16741=ADVANCED_FACE ( 'NONE', ( #13145 ), #11879, .T. ) ;
#16756=ORIENTED_EDGE ( 'NONE', *, *, #14537, .T. ) ;
#16759=CARTESIAN_POINT ( 'NONE',  ( 12.25209451496117197, 10.00000000000000000, 0.000000000000000000 ) ) ;
#16760=ORIENTED_EDGE ( 'NONE', *, *, #5239, .F. ) ;
#16761=ORIENTED_EDGE ( 'NONE', *, *, #18479, .F. ) ;
#16765=CARTESIAN_POINT ( 'NONE',  ( -1.437849085826860884, 16.00000000000000000, 1.000000000000000000 ) ) ;
#16768=CARTESIAN_POINT ( 'NONE',  ( 5.381197846483058989, -14.00000000000000000, 2.000000000000000000 ) ) ;
#16771=EDGE_CURVE ( 'NONE', #13229, #12054, #8449, .T. ) ;
#16772=CARTESIAN_POINT ( 'NONE',  ( -12.50209451496117197, 11.64110105645932691, 10.00000000000000000 ) ) ;
#16788=CARTESIAN_POINT ( 'NONE',  ( 23.31633994409548549, 11.64110105645932691, 0.000000000000000000 ) ) ;
#16790=CARTESIAN_POINT ( 'NONE',  ( -9.000000000000000000, -9.999999999999992895, 1.000000000000000000 ) ) ;
#16792=EDGE_LOOP ( 'NONE', ( #10613, #11541, #6535, #4852, #12103, #12268, #11712, #19580, #11609, #9791 ) ) ;
#16794=CYLINDRICAL_SURFACE ( 'NONE', #11010, 10.00000000000000000 ) ;
#16797=CARTESIAN_POINT ( 'NONE',  ( 27.00000000000000000, 0.000000000000000000, 1.000000000000000000 ) ) ;
#16802=CARTESIAN_POINT ( 'NONE',  ( -0.000000000000000000, 11.64110105645932691, 0.000000000000000000 ) ) ;
#16811=PLANE ( 'NONE',  #13649 ) ;
#16818=ORIENTED_EDGE ( 'NONE', *, *, #6030, .T. ) ;
#16819=CARTESIAN_POINT ( 'NONE',  ( -20.00349085826861995, 11.64110105645932691, 0.000000000000000000 ) ) ;
#16820=LINE ( 'NONE', #19971, #2594 ) ;
#16821=EDGE_CURVE ( 'NONE', #9770, #962, #2885, .T. ) ;
#16829=ORIENTED_EDGE ( 'NONE', *, *, #18241, .T. ) ;
#16836=ORIENTED_EDGE ( 'NONE', *, *, #5174, .F. ) ;
#16838=PLANE ( 'NONE',  #13957 ) ;
#16843=CARTESIAN_POINT ( 'NONE',  ( 0.000000000000000000, 11.64110105645932691, 10.00000000000000000 ) ) ;
#16846=DIRECTION ( 'NONE',  ( -0.000000000000000000, 0.000000000000000000, -1.000000000000000000 ) ) ;
#16857=ORIENTED_EDGE ( 'NONE', *, *, #12184, .F. ) ;
#16861=VERTEX_POINT ( 'NONE', #7594 ) ;
#16869=PLANE ( 'NONE',  #3474 ) ;
#16878=ADVANCED_FACE ( 'NONE', ( #2678 ), #8857, .T. ) ;
#16881=ORIENTED_EDGE ( 'NONE', *, *, #14969, .F. ) ;
#16888=VERTEX_POINT ( 'NONE', #15535 ) ;
#16891=ORIENTED_EDGE ( 'NONE', *, *, #594, .T. ) ;
#16892=CARTESIAN_POINT ( 'NONE',  ( 0.000000000000000000, 11.64110105645932691, 10.00000000000000000 ) ) ;
#16893=CARTESIAN_POINT ( 'NONE',  ( 0.000000000000000000, 11.64110105645932691, 10.00000000000000000 ) ) ;
#16896=LINE ( 'NONE', #2466, #3192 ) ;
#16898=DIRECTION ( 'NONE',  ( 0.000000000000000000, 1.000000000000000000, -0.000000000000000000 ) ) ;
#16899=DIRECTION ( 'NONE',  ( 1.000000000000000000, 0.000000000000000000, 0.000000000000000000 ) ) ;
#16911=CARTESIAN_POINT ( 'NONE',  ( 14.31494360078803041, 10.00000000000000000, 1.000000000000000000 ) ) ;
#16912=ORIENTED_EDGE ( 'NONE', *, *, #14969, .T. ) ;
#16916=ORIENTED_EDGE ( 'NONE', *, *, #1860, .T. ) ;
#16917=DIRECTION ( 'NONE',  ( 1.000000000000000000, 0.000000000000000000, 0.000000000000000000 ) ) ;
#16918=DIRECTION ( 'NONE',  ( 1.000000000000000000, 0.000000000000000000, 0.000000000000000000 ) ) ;
#16922=CARTESIAN_POINT ( 'NONE',  ( -22.81633994409548549, 10.00000000000000000, 0.000000000000000000 ) ) ;
#16934=ORIENTED_EDGE ( 'NONE', *, *, #8787, .T. ) ;
#16938=ORIENTED_EDGE ( 'NONE', *, *, #15013, .T. ) ;
#16940=ORIENTED_EDGE ( 'NONE', *, *, #690, .F. ) ;
#16942=CARTESIAN_POINT ( 'NONE',  ( -5.563547257480587760, 0.000000000000000000, 1.000000000000000000 ) ) ;
#16945=LINE ( 'NONE', #17161, #9727 ) ;
#16949=ADVANCED_FACE ( 'NONE', ( #18794 ), #18483, .T. ) ;
#16950=ADVANCED_FACE ( 'NONE', ( #17208 ), #14067, .T. ) ;
#16957=DIRECTION ( 'NONE',  ( -1.000000000000000000, 0.000000000000000000, 0.000000000000000000 ) ) ;
#16958=ORIENTED_EDGE ( 'NONE', *, *, #3849, .T. ) ;
#16968=COLOUR_RGB ( '', 0.72549020, 0.75294118, 0.79215686) ;
#16971=PLANE ( 'NONE',  #7489 ) ;
#16973=CYLINDRICAL_SURFACE ( 'NONE', #14406, 1.499999999999999556 ) ;
#16974=LINE ( 'NONE', #2650, #13309 ) ;
#16979=DIRECTION ( 'NONE',  ( -1.040834085586084454E-15, 1.000000000000000000, 8.673617379884037444E-16 ) ) ;
#16985=CIRCLE ( 'NONE', #3967, 2.999999999999999112 ) ;
#16990=ORIENTED_EDGE ( 'NONE', *, *, #9361, .F. ) ;
#16994=VERTEX_POINT ( 'NONE', #16797 ) ;
#16997=EDGE_CURVE ( 'NONE', #17851, #18752, #16896, .T. ) ;
#16998=AXIS2_PLACEMENT_3D ( 'NONE', #15966, #11073, #10867 ) ;
#17000=VECTOR ( 'NONE', #13644, 1000.000000000000000 ) ;
#17011=ORIENTED_EDGE ( 'NONE', *, *, #5509, .F. ) ;
#17014=ORIENTED_EDGE ( 'NONE', *, *, #10117, .T. ) ;
#17015=CARTESIAN_POINT ( 'NONE',  ( -6.313547257480587760, 10.00000000000000000, 1.000000000000000000 ) ) ;
#17017=VERTEX_POINT ( 'NONE', #7397 ) ;
#17020=ORIENTED_EDGE ( 'NONE', *, *, #14205, .T. ) ;
#17021=CARTESIAN_POINT ( 'NONE',  ( 10.18924542913430820, 16.00000000000000000, 1.000000000000000000 ) ) ;
#17022=DIRECTION ( 'NONE',  ( -0.000000000000000000, -0.000000000000000000, -1.000000000000000000 ) ) ;
#17023=AXIS2_PLACEMENT_3D ( 'NONE', #12757, #20526, #9314 ) ;
#17026=DIRECTION ( 'NONE',  ( 0.000000000000000000, 1.000000000000000000, -0.000000000000000000 ) ) ;
#17034=STYLED_ITEM ( 'NONE', ( #16326 ), #4314 ) ;
#17036=PLANE ( 'NONE',  #9615 ) ;
#17037=CARTESIAN_POINT ( 'NONE',  ( -3.500698171653725765, 10.00000000000000000, 1.000000000000000000 ) ) ;
#17047=ORIENTED_EDGE ( 'NONE', *, *, #9956, .T. ) ;
#17048=CARTESIAN_POINT ( 'NONE',  ( -11.75209451496117197, 0.000000000000000000, 1.000000000000000000 ) ) ;
#17051=PLANE ( 'NONE',  #8600 ) ;
#17057=CARTESIAN_POINT ( 'NONE',  ( -4.250698171653726654, 0.000000000000000000, 1.000000000000000000 ) ) ;
#17065=ORIENTED_EDGE ( 'NONE', *, *, #7735, .T. ) ;
#17069=ORIENTED_EDGE ( 'NONE', *, *, #18190, .F. ) ;
#17070=VECTOR ( 'NONE', #3684, 1000.000000000000000 ) ;
#17072=ORIENTED_EDGE ( 'NONE', *, *, #20684, .F. ) ;
#17077=LINE ( 'NONE', #19923, #5974 ) ;
#17087=ORIENTED_EDGE ( 'NONE', *, *, #4237, .F. ) ;
#17093=VERTEX_POINT ( 'NONE', #9471 ) ;
#17099=ORIENTED_EDGE ( 'NONE', *, *, #20443, .T. ) ;
#17104=CARTESIAN_POINT ( 'NONE',  ( -15.00000000000000000, -6.000000000000000000, 1.000000000000000000 ) ) ;
#17106=FACE_OUTER_BOUND ( 'NONE', #16404, .T. ) ;
#17108=DIRECTION ( 'NONE',  ( 1.000000000000000000, 0.000000000000000000, -0.000000000000000000 ) ) ;
#17111=DIRECTION ( 'NONE',  ( 1.000000000000000000, 0.000000000000000000, -0.000000000000000000 ) ) ;
#17116=VECTOR ( 'NONE', #19408, 1000.000000000000000 ) ;
#17117=EDGE_CURVE ( 'NONE', #16861, #682, #10543, .T. ) ;
#17129=DIRECTION ( 'NONE',  ( 0.000000000000000000, 0.000000000000000000, -1.000000000000000000 ) ) ;
#17133=LINE ( 'NONE', #10869, #18945 ) ;
#17157=DIRECTION ( 'NONE',  ( 0.000000000000000000, -1.000000000000000000, 0.000000000000000000 ) ) ;
#17158=VECTOR ( 'NONE', #5495, 1000.000000000000000 ) ;
#17161=CARTESIAN_POINT ( 'NONE',  ( -1.437849085826860884, 0.000000000000000000, 0.000000000000000000 ) ) ;
#17167=VECTOR ( 'NONE', #10500, 1000.000000000000000 ) ;
#17168=EDGE_CURVE ( 'NONE', #6657, #1638, #1730, .T. ) ;
#17171=ORIENTED_EDGE ( 'NONE', *, *, #11899, .T. ) ;
#17174=ORIENTED_EDGE ( 'NONE', *, *, #19240, .T. ) ;
#17176=CARTESIAN_POINT ( 'NONE',  ( 0.000000000000000000, 10.00000000000000000, 1.000000000000000000 ) ) ;
#17178=CARTESIAN_POINT ( 'NONE',  ( -24.87918902992234393, 16.00000000000000000, 1.000000000000000000 ) ) ;
#17187=VERTEX_POINT ( 'NONE', #251 ) ;
#17189=DIRECTION ( 'NONE',  ( -0.000000000000000000, -0.000000000000000000, -1.000000000000000000 ) ) ;
#17190=EDGE_CURVE ( 'NONE', #17093, #6020, #6542, .T. ) ;
#17193=ORIENTED_EDGE ( 'NONE', *, *, #4835, .F. ) ;
#17199=CARTESIAN_POINT ( 'NONE',  ( -12.50209451496117197, 0.000000000000000000, 1.000000000000000000 ) ) ;
#17208=FACE_OUTER_BOUND ( 'NONE', #3670, .T. ) ;
#17210=FACE_OUTER_BOUND ( 'NONE', #12542, .T. ) ;
#17211=CARTESIAN_POINT ( 'NONE',  ( -22.06633994409548194, 16.00000000000000000, 1.000000000000000000 ) ) ;
#17218=EDGE_LOOP ( 'NONE', ( #7226, #8895, #7117, #19848 ) ) ;
#17222=ORIENTED_EDGE ( 'NONE', *, *, #12397, .T. ) ;
#17224=VERTEX_POINT ( 'NONE', #7805 ) ;
#17228=DIRECTION ( 'NONE',  ( -1.000000000000000000, 0.000000000000000000, 0.000000000000000000 ) ) ;
#17230=CARTESIAN_POINT ( 'NONE',  ( 0.000000000000000000, 16.00000000000000000, 1.000000000000000000 ) ) ;
#17236=DIRECTION ( 'NONE',  ( 1.000000000000000000, 0.000000000000000000, 0.000000000000000000 ) ) ;
#17251=CARTESIAN_POINT ( 'NONE',  ( 12.25209451496117197, 16.00000000000000000, 1.000000000000000000 ) ) ;
#17254=VECTOR ( 'NONE', #662, 1000.000000000000000 ) ;
#17255=EDGE_CURVE ( 'NONE', #3633, #19354, #1520, .T. ) ;
#17256=FACE_OUTER_BOUND ( 'NONE', #19154, .T. ) ;
#17268=ORIENTED_EDGE ( 'NONE', *, *, #12976, .T. ) ;
#17269=ORIENTED_EDGE ( 'NONE', *, *, #2132, .T. ) ;
#17270=DIRECTION ( 'NONE',  ( 1.000000000000000000, -0.000000000000000000, 0.000000000000000000 ) ) ;
#17275=FACE_OUTER_BOUND ( 'NONE', #19674, .T. ) ;
#17278=CARTESIAN_POINT ( 'NONE',  ( -26.19203811574920593, 10.00000000000000000, 1.000000000000000000 ) ) ;
#17283=ORIENTED_EDGE ( 'NONE', *, *, #17255, .F. ) ;
#17293=ORIENTED_EDGE ( 'NONE', *, *, #4575, .T. ) ;
#17294=EDGE_CURVE ( 'NONE', #8687, #13997, #8720, .T. ) ;
#17296=DIRECTION ( 'NONE',  ( 1.000000000000000000, 0.000000000000000000, 0.000000000000000000 ) ) ;
#17298=CARTESIAN_POINT ( 'NONE',  ( 0.000000000000000000, 10.00000000000000000, 1.000000000000000000 ) ) ;
#17301=ORIENTED_EDGE ( 'NONE', *, *, #8511, .T. ) ;
#17305=DIRECTION ( 'NONE',  ( -1.000000000000000000, 0.000000000000000000, 0.000000000000000000 ) ) ;
#17309=DIRECTION ( 'NONE',  ( -0.000000000000000000, -0.000000000000000000, -1.000000000000000000 ) ) ;
#17311=CARTESIAN_POINT ( 'NONE',  ( -9.000000000000000000, -9.999999999999992895, 2.000000000000000000 ) ) ;
#17316=AXIS2_PLACEMENT_3D ( 'NONE', #15510, #18769, #2862 ) ;
#17317=ORIENTED_EDGE ( 'NONE', *, *, #13846, .T. ) ;
#17320=ORIENTED_EDGE ( 'NONE', *, *, #9473, .T. ) ;
#17321=VECTOR ( 'NONE', #15651, 1000.000000000000000 ) ;
#17322=ADVANCED_FACE ( 'NONE', ( #17928 ), #13421, .T. ) ;
#17324=ORIENTED_EDGE ( 'NONE', *, *, #19763, .T. ) ;
#17331=EDGE_CURVE ( 'NONE', #13057, #18061, #11646, .T. ) ;
#17335=DIRECTION ( 'NONE',  ( 0.000000000000000000, 1.000000000000000000, 0.000000000000000000 ) ) ;
#17340=CARTESIAN_POINT ( 'NONE',  ( 0.000000000000000000, 0.000000000000000000, 1.000000000000000000 ) ) ;
#17342=ORIENTED_EDGE ( 'NONE', *, *, #8352, .F. ) ;
#17346=AXIS2_PLACEMENT_3D ( 'NONE', #15197, #20447, #4216 ) ;
#17354=ORIENTED_EDGE ( 'NONE', *, *, #16387, .T. ) ;
#17358=DIRECTION ( 'NONE',  ( 0.000000000000000000, 1.000000000000000000, -0.000000000000000000 ) ) ;
#17366=VECTOR ( 'NONE', #10553, 1000.000000000000000 ) ;
#17368=CARTESIAN_POINT ( 'NONE',  ( -10.43924542913431175, 10.00000000000000000, 1.000000000000000000 ) ) ;
#17369=EDGE_CURVE ( 'NONE', #19920, #19324, #3499, .T. ) ;
#17385=CARTESIAN_POINT ( 'NONE',  ( -22.06633994409548194, 10.00000000000000000, 1.000000000000000000 ) ) ;
#17386=FACE_OUTER_BOUND ( 'NONE', #939, .T. ) ;
#17387=CARTESIAN_POINT ( 'NONE',  ( 15.00000000000000355, -5.999999999999996447, 2.000000000000000000 ) ) ;
#17400=ORIENTED_EDGE ( 'NONE', *, *, #16821, .T. ) ;
#17401=VECTOR ( 'NONE', #2113, 1000.000000000000000 ) ;
#17403=VECTOR ( 'NONE', #19323, 1000.000000000000000 ) ;
#17406=ORIENTED_EDGE ( 'NONE', *, *, #784, .F. ) ;
#17407=EDGE_CURVE ( 'NONE', #12358, #5810, #11068, .T. ) ;
#17411=EDGE_CURVE ( 'NONE', #13991, #9844, #14685, .T. ) ;
#17421=CYLINDRICAL_SURFACE ( 'NONE', #7439, 10.00000000000000000 ) ;
#17423=CARTESIAN_POINT ( 'NONE',  ( 26.69203811574920948, 1.543443504701929706E-14, 1.000000000000000000 ) ) ;
#17429=ORIENTED_EDGE ( 'NONE', *, *, #1493, .F. ) ;
#17432=ORIENTED_EDGE ( 'NONE', *, *, #8787, .F. ) ;
#17433=AXIS2_PLACEMENT_3D ( 'NONE', #12630, #19035, #4690 ) ;
#17437=DIRECTION ( 'NONE',  ( -1.000000000000000000, 0.000000000000000000, 0.000000000000000000 ) ) ;
#17438=ORIENTED_EDGE ( 'NONE', *, *, #669, .T. ) ;
#17444=AXIS2_PLACEMENT_3D ( 'NONE', #17298, #6018, #18786 ) ;
#17445=SURFACE_SIDE_STYLE ('',( #13043 ) ) ;
#17447=CARTESIAN_POINT ( 'NONE',  ( 19.19064177244175440, 16.00000000000000000, 1.000000000000000000 ) ) ;
#17451=LINE ( 'NONE', #6479, #19447 ) ;
#17453=ORIENTED_EDGE ( 'NONE', *, *, #18102, .T. ) ;
#17457=EDGE_CURVE ( 'NONE', #17224, #17017, #11818, .T. ) ;
#17462=ADVANCED_FACE ( 'NONE', ( #3908 ), #16971, .F. ) ;
#17466=DIRECTION ( 'NONE',  ( 1.000000000000000000, 0.000000000000000000, 0.000000000000000000 ) ) ;
#17479=ORIENTED_EDGE ( 'NONE', *, *, #2061, .T. ) ;
#17481=DIRECTION ( 'NONE',  ( 1.000000000000000000, 0.000000000000000000, -0.000000000000000000 ) ) ;
#17482=VERTEX_POINT ( 'NONE', #2539 ) ;
#17484=FACE_OUTER_BOUND ( 'NONE', #18076, .T. ) ;
#17488=ADVANCED_FACE ( 'NONE', ( #12263 ), #16869, .T. ) ;
#17500=ORIENTED_EDGE ( 'NONE', *, *, #17331, .T. ) ;
#17504=ORIENTED_EDGE ( 'NONE', *, *, #17255, .T. ) ;
#17506=CARTESIAN_POINT ( 'NONE',  ( 0.000000000000000000, 16.00000000000000000, 1.000000000000000000 ) ) ;
#17515=EDGE_CURVE ( 'NONE', #6665, #11041, #20134, .T. ) ;
#17516=CARTESIAN_POINT ( 'NONE',  ( -27.94203811574921659, 9.999999999999998224, 0.000000000000000000 ) ) ;
#17519=DIRECTION ( 'NONE',  ( 1.000000000000000000, 0.000000000000000000, -0.000000000000000000 ) ) ;
#17530=ADVANCED_FACE ( 'NONE', ( #8928 ), #1190, .T. ) ;
#17532=CARTESIAN_POINT ( 'NONE',  ( 27.44203811574919882, 11.64110105645932691, 10.00000000000000000 ) ) ;
#17538=CARTESIAN_POINT ( 'NONE',  ( -29.44326362367960570, 13.15740888934567465, -1.641876399273490883E-15 ) ) ;
#17539=VECTOR ( 'NONE', #4092, 1000.000000000000000 ) ;
#17546=CARTESIAN_POINT ( 'NONE',  ( 0.000000000000000000, 16.00000000000000000, 1.000000000000000000 ) ) ;
#17548=ORIENTED_EDGE ( 'NONE', *, *, #2193, .T. ) ;
#17557=VERTEX_POINT ( 'NONE', #15507 ) ;
#17558=CARTESIAN_POINT ( 'NONE',  ( 14.99999999999999645, 3.000000000000003553, 1.000000000000000000 ) ) ;
#17559=VECTOR ( 'NONE', #4473, 1000.000000000000000 ) ;
#17570=CARTESIAN_POINT ( 'NONE',  ( -13.81494360078803396, 10.00000000000000000, 1.000000000000000000 ) ) ;
#17581=CARTESIAN_POINT ( 'NONE',  ( 0.000000000000000000, 11.64110105645932691, 10.00000000000000000 ) ) ;
#17584=ORIENTED_EDGE ( 'NONE', *, *, #18190, .T. ) ;
#17586=AXIS2_PLACEMENT_3D ( 'NONE', #8109, #12899, #19304 ) ;
#17605=EDGE_LOOP ( 'NONE', ( #15451, #9352, #16172, #8580 ) ) ;
#17612=LINE ( 'NONE', #14473, #8763 ) ;
#17631=ORIENTED_EDGE ( 'NONE', *, *, #11501, .F. ) ;
#17644=LINE ( 'NONE', #3528, #15971 ) ;
#17646=DIRECTION ( 'NONE',  ( 0.000000000000000000, -1.000000000000000000, 0.000000000000000000 ) ) ;
#17648=DIRECTION ( 'NONE',  ( 0.000000000000000000, -1.000000000000000000, 0.000000000000000000 ) ) ;
#17653=DIRECTION ( 'NONE',  ( 1.000000000000000000, 0.000000000000000000, 0.000000000000000000 ) ) ;
#17655=ORIENTED_EDGE ( 'NONE', *, *, #6466, .F. ) ;
#17659=VECTOR ( 'NONE', #13618, 1000.000000000000000 ) ;
#17660=CARTESIAN_POINT ( 'NONE',  ( -20.75349085826862350, 11.64110105645932691, 0.000000000000000000 ) ) ;
#17663=EDGE_CURVE ( 'NONE', #193, #17482, #16700, .T. ) ;
#17664=VECTOR ( 'NONE', #162, 1000.000000000000000 ) ;
#17667=VERTEX_POINT ( 'NONE', #11219 ) ;
#17671=CARTESIAN_POINT ( 'NONE',  ( -15.00000000000000000, -6.000000000000000000, 2.000000000000000000 ) ) ;
#17681=VECTOR ( 'NONE', #5419, 1000.000000000000000 ) ;
#17687=VERTEX_POINT ( 'NONE', #18869 ) ;
#17690=FACE_OUTER_BOUND ( 'NONE', #9460, .T. ) ;
#17699=LINE ( 'NONE', #17385, #4673 ) ;
#17701=DIRECTION ( 'NONE',  ( -0.9848077530122082424, -0.1736481776669292765, 0.000000000000000000 ) ) ;
#17708=AXIS2_PLACEMENT_3D ( 'NONE', #19926, #2440, #136 ) ;
#17710=VECTOR ( 'NONE', #5633, 1000.000000000000000 ) ;
#17712=DIRECTION ( 'NONE',  ( 0.000000000000000000, -0.000000000000000000, 1.000000000000000000 ) ) ;
#17715=MECHANICAL_DESIGN_GEOMETRIC_PRESENTATION_REPRESENTATION('',(#17034),#1002);
#17716=ORIENTED_EDGE ( 'NONE', *, *, #227, .F. ) ;
#17720=EDGE_LOOP ( 'NONE', ( #20602, #12661, #17438, #19535 ) ) ;
#17721=CIRCLE ( 'NONE', #8031, 10.00000000000000000 ) ;
#17726=CARTESIAN_POINT ( 'NONE',  ( -0.000000000000000000, 11.64110105645932691, 0.000000000000000000 ) ) ;
#17727=ORIENTED_EDGE ( 'NONE', *, *, #12184, .T. ) ;
#17729=CARTESIAN_POINT ( 'NONE',  ( -5.381197846483055436, -14.00000000000000000, 1.000000000000000000 ) ) ;
#17735=CIRCLE ( 'NONE', #4040, 10.00000000000000000 ) ;
#17739=AXIS2_PLACEMENT_3D ( 'NONE', #3681, #3788, #11730 ) ;
#17747=ORIENTED_EDGE ( 'NONE', *, *, #13376, .T. ) ;
#17752=AXIS2_PLACEMENT_3D ( 'NONE', #9854, #2213, #14868 ) ;
#17753=ORIENTED_EDGE ( 'NONE', *, *, #15092, .F. ) ;
#17755=LINE ( 'NONE', #3523, #11332 ) ;
#17764=VECTOR ( 'NONE', #2290, 1000.000000000000000 ) ;
#17770=DIRECTION ( 'NONE',  ( 0.000000000000000000, -1.000000000000000000, 0.000000000000000000 ) ) ;
#17772=ORIENTED_EDGE ( 'NONE', *, *, #9871, .T. ) ;
#17791=CIRCLE ( 'NONE', #13113, 1.499999999999996225 ) ;
#17799=DIRECTION ( 'NONE',  ( -1.000000000000000000, 0.000000000000000000, 0.000000000000000000 ) ) ;
#17801=EDGE_LOOP ( 'NONE', ( #16829, #9349, #14836, #4778 ) ) ;
#17805=LINE ( 'NONE', #336, #19231 ) ;
#17814=CYLINDRICAL_SURFACE ( 'NONE', #691, 10.00000000000000000 ) ;
#17815=ORIENTED_EDGE ( 'NONE', *, *, #14037, .F. ) ;
#17817=CARTESIAN_POINT ( 'NONE',  ( -1.437849085826860884, 10.00000000000000000, 1.000000000000000000 ) ) ;
#17824=ORIENTED_EDGE ( 'NONE', *, *, #4112, .F. ) ;
#17825=ORIENTED_EDGE ( 'NONE', *, *, #13312, .T. ) ;
#17826=FACE_OUTER_BOUND ( 'NONE', #5439, .T. ) ;
#17827=EDGE_CURVE ( 'NONE', #3742, #13535, #17133, .T. ) ;
#17828=DIRECTION ( 'NONE',  ( -1.000000000000000000, 0.000000000000000000, 0.000000000000000000 ) ) ;
#17834=EDGE_CURVE ( 'NONE', #13339, #7911, #7729, .T. ) ;
#17839=DIRECTION ( 'NONE',  ( -0.000000000000000000, -0.000000000000000000, -1.000000000000000000 ) ) ;
#17840=VERTEX_POINT ( 'NONE', #15073 ) ;
#17844=VERTEX_POINT ( 'NONE', #13504 ) ;
#17847=CARTESIAN_POINT ( 'NONE',  ( 7.500000000000002665, -9.999999999999991118, 1.000000000000000000 ) ) ;
#17848=ORIENTED_EDGE ( 'NONE', *, *, #3079, .T. ) ;
#17849=ORIENTED_EDGE ( 'NONE', *, *, #6084, .F. ) ;
#17851=VERTEX_POINT ( 'NONE', #7618 ) ;
#17854=ORIENTED_EDGE ( 'NONE', *, *, #9045, .T. ) ;
#17868=ORIENTED_EDGE ( 'NONE', *, *, #4669, .F. ) ;
#17873=ORIENTED_EDGE ( 'NONE', *, *, #3743, .T. ) ;
#17875=CARTESIAN_POINT ( 'NONE',  ( 0.000000000000000000, 0.000000000000000000, 1.000000000000000000 ) ) ;
#17876=VECTOR ( 'NONE', #12982, 1000.000000000000000 ) ;
#17881=AXIS2_PLACEMENT_3D ( 'NONE', #18686, #17108, #4246 ) ;
#17889=DIRECTION ( 'NONE',  ( 0.000000000000000000, -1.000000000000000000, 0.000000000000000000 ) ) ;
#17897=FILL_AREA_STYLE ('',( #6606 ) ) ;
#17899=DIRECTION ( 'NONE',  ( -1.000000000000000000, 0.000000000000000000, 0.000000000000000000 ) ) ;
#17903=CARTESIAN_POINT ( 'NONE',  ( 15.06494360078803041, 0.000000000000000000, 1.000000000000000000 ) ) ;
#17912=DIRECTION ( 'NONE',  ( 1.000000000000000000, 0.000000000000000000, 0.000000000000000000 ) ) ;
#17915=EDGE_LOOP ( 'NONE', ( #12123, #15682, #4133, #18839 ) ) ;
#17919=VERTEX_POINT ( 'NONE', #9397 ) ;
#17923=LINE ( 'NONE', #771, #1569 ) ;
#17926=CARTESIAN_POINT ( 'NONE',  ( 23.31633994409548549, 0.000000000000000000, 1.000000000000000000 ) ) ;
#17928=FACE_OUTER_BOUND ( 'NONE', #12975, .T. ) ;
#17937=EDGE_CURVE ( 'NONE', #6555, #4233, #8144, .T. ) ;
#17940=ORIENTED_EDGE ( 'NONE', *, *, #16276, .T. ) ;
#17943=ORIENTED_EDGE ( 'NONE', *, *, #17411, .F. ) ;
#17944=VERTEX_POINT ( 'NONE', #3429 ) ;
#17945=LINE ( 'NONE', #14594, #18761 ) ;
#17949=AXIS2_PLACEMENT_3D ( 'NONE', #6795, #7105, #5427 ) ;
#17956=DIRECTION ( 'NONE',  ( 0.000000000000000000, 1.000000000000000000, -0.000000000000000000 ) ) ;
#17958=CARTESIAN_POINT ( 'NONE',  ( -8.376396343307449754, 0.000000000000000000, 1.000000000000000000 ) ) ;
#17966=VECTOR ( 'NONE', #5934, 1000.000000000000000 ) ;
#17968=LINE ( 'NONE', #13055, #3645 ) ;
#17975=EDGE_CURVE ( 'NONE', #20454, #10227, #3220, .T. ) ;
#17980=LINE ( 'NONE', #8471, #13805 ) ;
#17989=CARTESIAN_POINT ( 'NONE',  ( -18.69064177244175795, 0.000000000000000000, 1.000000000000000000 ) ) ;
#17995=ORIENTED_EDGE ( 'NONE', *, *, #15201, .F. ) ;
#18000=CARTESIAN_POINT ( 'NONE',  ( 14.31494360078803041, 11.64110105645932691, 10.00000000000000000 ) ) ;
#18004=AXIS2_PLACEMENT_3D ( 'NONE', #14286, #17335, #6362 ) ;
#18006=LINE ( 'NONE', #3676, #17876 ) ;
#18009=DIRECTION ( 'NONE',  ( 1.000000000000000000, 0.000000000000000000, 0.000000000000000000 ) ) ;
#18016=CARTESIAN_POINT ( 'NONE',  ( -8.376396343307449754, 0.000000000000000000, 1.000000000000000000 ) ) ;
#18020=ORIENTED_EDGE ( 'NONE', *, *, #5268, .T. ) ;
#18029=EDGE_CURVE ( 'NONE', #2724, #13538, #15969, .T. ) ;
#18032=DIRECTION ( 'NONE',  ( 0.000000000000000000, -1.000000000000000000, 0.000000000000000000 ) ) ;
#18033=LINE ( 'NONE', #7158, #16348 ) ;
#18035=DIRECTION ( 'NONE',  ( 1.000000000000000000, 0.000000000000000000, 0.000000000000000000 ) ) ;
#18038=CARTESIAN_POINT ( 'NONE',  ( 24.62918902992234038, 10.00000000000000000, 0.000000000000000000 ) ) ;
#18039=AXIS2_PLACEMENT_3D ( 'NONE', #1793, #16229, #8180 ) ;
#18043=ORIENTED_EDGE ( 'NONE', *, *, #5779, .T. ) ;
#18044=MANIFOLD_SOLID_BREP ( 'Boss-Extrude2', #4618 ) ;
#18052=LINE ( 'NONE', #9993, #5040 ) ;
#18053=ORIENTED_EDGE ( 'NONE', *, *, #3079, .F. ) ;
#18054=VERTEX_POINT ( 'NONE', #9498 ) ;
#18061=VERTEX_POINT ( 'NONE', #3736 ) ;
#18065=VECTOR ( 'NONE', #19582, 1000.000000000000000 ) ;
#18072=PLANE ( 'NONE',  #855 ) ;
#18076=EDGE_LOOP ( 'NONE', ( #8639, #9084, #717, #3076 ) ) ;
#18080=ORIENTED_EDGE ( 'NONE', *, *, #8813, .F. ) ;
#18085=EDGE_LOOP ( 'NONE', ( #19944, #11473, #10204, #2243 ) ) ;
#18091=PLANE ( 'NONE',  #13986 ) ;
#18094=CARTESIAN_POINT ( 'NONE',  ( 0.000000000000000000, 10.00000000000000000, 1.000000000000000000 ) ) ;
#18096=AXIS2_PLACEMENT_3D ( 'NONE', #12264, #4326, #5999 ) ;
#18098=LINE ( 'NONE', #10141, #19387 ) ;
#18102=EDGE_CURVE ( 'NONE', #12575, #5162, #7087, .T. ) ;
#18103=EDGE_CURVE ( 'NONE', #10774, #1441, #13650, .T. ) ;
#18104=CARTESIAN_POINT ( 'NONE',  ( 19.19064177244175440, 11.64110105645932691, 10.00000000000000000 ) ) ;
#18105=CARTESIAN_POINT ( 'NONE',  ( 8.876396343307449754, 0.000000000000000000, 0.000000000000000000 ) ) ;
#18109=EDGE_CURVE ( 'NONE', #9991, #10193, #6621, .T. ) ;
#18113=EDGE_LOOP ( 'NONE', ( #2155, #7167, #2773, #15143 ) ) ;
#18114=VECTOR ( 'NONE', #8576, 1000.000000000000000 ) ;
#18116=CARTESIAN_POINT ( 'NONE',  ( -15.00000000000000000, 0.000000000000000000, 1.000000000000000000 ) ) ;
#18125=FACE_OUTER_BOUND ( 'NONE', #18085, .T. ) ;
#18135=LINE ( 'NONE', #1079, #4005 ) ;
#18137=ORIENTED_EDGE ( 'NONE', *, *, #14774, .F. ) ;
#18141=DIRECTION ( 'NONE',  ( -0.000000000000000000, -0.000000000000000000, -1.000000000000000000 ) ) ;
#18142=CARTESIAN_POINT ( 'NONE',  ( -26.19203811574920593, 11.64110105645932691, 10.00000000000000000 ) ) ;
#18155=ORIENTED_EDGE ( 'NONE', *, *, #18029, .T. ) ;
#18157=FACE_OUTER_BOUND ( 'NONE', #18113, .T. ) ;
#18162=DIRECTION ( 'NONE',  ( 0.000000000000000000, 0.000000000000000000, 1.000000000000000000 ) ) ;
#18163=ORIENTED_EDGE ( 'NONE', *, *, #9871, .F. ) ;
#18187=ORIENTED_EDGE ( 'NONE', *, *, #8397, .F. ) ;
#18188=LINE ( 'NONE', #16598, #1637 ) ;
#18190=EDGE_CURVE ( 'NONE', #20631, #6657, #14916, .T. ) ;
#18197=EDGE_CURVE ( 'NONE', #4996, #4809, #2943, .T. ) ;
#18198=EDGE_CURVE ( 'NONE', #2900, #6116, #8451, .T. ) ;
#18211=DIRECTION ( 'NONE',  ( -0.000000000000000000, -0.000000000000000000, -1.000000000000000000 ) ) ;
#18214=DIRECTION ( 'NONE',  ( 0.000000000000000000, -0.000000000000000000, 1.000000000000000000 ) ) ;
#18226=FACE_OUTER_BOUND ( 'NONE', #17218, .T. ) ;
#18228=EDGE_CURVE ( 'NONE', #2639, #12514, #20061, .T. ) ;
#18231=VERTEX_POINT ( 'NONE', #14169 ) ;
#18239=LINE ( 'NONE', #19822, #10256 ) ;
#18240=ADVANCED_FACE ( 'NONE', ( #17210 ), #13962, .T. ) ;
#18241=EDGE_CURVE ( 'NONE', #12822, #14996, #14070, .T. ) ;
#18242=PLANE ( 'NONE',  #14655 ) ;
#18251=EDGE_LOOP ( 'NONE', ( #8462, #17099, #2672, #4367 ) ) ;
#18255=ADVANCED_FACE ( 'NONE', ( #7596 ), #7807, .T. ) ;
#18257=ORIENTED_EDGE ( 'NONE', *, *, #15201, .T. ) ;
#18259=PLANE ( 'NONE',  #8047 ) ;
#18261=ORIENTED_EDGE ( 'NONE', *, *, #1314, .F. ) ;
#18265=EDGE_LOOP ( 'NONE', ( #8741, #17174, #5786, #17825 ) ) ;
#18267=CARTESIAN_POINT ( 'NONE',  ( 19.19064177244175440, 10.00000000000000000, 1.000000000000000000 ) ) ;
#18286=EDGE_LOOP ( 'NONE', ( #11859, #527, #17011, #12694 ) ) ;
#18288=ORIENTED_EDGE ( 'NONE', *, *, #3250, .F. ) ;
#18289=DIRECTION ( 'NONE',  ( 1.000000000000000000, 0.000000000000000000, 0.000000000000000000 ) ) ;
#18293=CARTESIAN_POINT ( 'NONE',  ( -30.80549002841696193, 5.431839045955507927, 1.000000000000000000 ) ) ;
#18301=FACE_OUTER_BOUND ( 'NONE', #15392, .T. ) ;
#18306=EDGE_LOOP ( 'NONE', ( #10878, #7223, #12936, #17020 ) ) ;
#18307=VERTEX_POINT ( 'NONE', #7400 ) ;
#18311=ORIENTED_EDGE ( 'NONE', *, *, #14452, .T. ) ;
#18317=VECTOR ( 'NONE', #2693, 1000.000000000000000 ) ;
#18328=VECTOR ( 'NONE', #17309, 1000.000000000000000 ) ;
#18329=CARTESIAN_POINT ( 'NONE',  ( 0.6250000000000005551, 10.00000000000000000, 1.000000000000000000 ) ) ;
#18338=DIRECTION ( 'NONE',  ( 0.000000000000000000, -1.000000000000000000, 0.000000000000000000 ) ) ;
#18340=ORIENTED_EDGE ( 'NONE', *, *, #16252, .F. ) ;
#18341=CARTESIAN_POINT ( 'NONE',  ( 9.000000000000000000, -9.999999999999991118, 2.000000000000000000 ) ) ;
#18342=VECTOR ( 'NONE', #14682, 1000.000000000000000 ) ;
#18345=VECTOR ( 'NONE', #4374, 1000.000000000000000 ) ;
#18348=PLANE ( 'NONE',  #19363 ) ;
#18351=FACE_OUTER_BOUND ( 'NONE', #16042, .T. ) ;
#18354=AXIS2_PLACEMENT_3D ( 'NONE', #9804, #9903, #392 ) ;
#18360=EDGE_CURVE ( 'NONE', #5953, #5929, #7500, .T. ) ;
#18363=AXIS2_PLACEMENT_3D ( 'NONE', #2404, #19888, #525 ) ;
#18365=EDGE_CURVE ( 'NONE', #13057, #15932, #20263, .T. ) ;
#18367=CARTESIAN_POINT ( 'NONE',  ( -22.81633994409548549, 0.000000000000000000, 1.000000000000000000 ) ) ;
#18368=ORIENTED_EDGE ( 'NONE', *, *, #11213, .T. ) ;
#18370=LINE ( 'NONE', #10615, #8148 ) ;
#18372=VERTEX_POINT ( 'NONE', #2994 ) ;
#18373=CARTESIAN_POINT ( 'NONE',  ( -27.00000000000000000, 0.000000000000000000, 0.000000000000000000 ) ) ;
#18376=EDGE_CURVE ( 'NONE', #3058, #17557, #9166, .T. ) ;
#18377=FACE_OUTER_BOUND ( 'NONE', #13769, .T. ) ;
#18383=AXIS2_PLACEMENT_3D ( 'NONE', #8369, #11398, #5434 ) ;
#18390=ORIENTED_EDGE ( 'NONE', *, *, #10873, .F. ) ;
#18395=CARTESIAN_POINT ( 'NONE',  ( -9.000000000000000000, -9.999999999999992895, 1.000000000000000000 ) ) ;
#18398=AXIS2_PLACEMENT_3D ( 'NONE', #19614, #9536, #7964 ) ;
#18399=VERTEX_POINT ( 'NONE', #10942 ) ;
#18402=DIRECTION ( 'NONE',  ( 0.000000000000000000, -1.000000000000000000, 0.000000000000000000 ) ) ;
#18404=DIRECTION ( 'NONE',  ( 1.000000000000000000, 0.000000000000000000, -0.000000000000000000 ) ) ;
#18405=DIRECTION ( 'NONE',  ( -0.9848077530122080203, 0.1736481776669309696, 0.000000000000000000 ) ) ;
#18419=ORIENTED_EDGE ( 'NONE', *, *, #15555, .F. ) ;
#18421=CARTESIAN_POINT ( 'NONE',  ( 2.687849085826861995, 10.00000000000000000, 1.000000000000000000 ) ) ;
#18424=FACE_OUTER_BOUND ( 'NONE', #9512, .T. ) ;
#18425=CARTESIAN_POINT ( 'NONE',  ( 0.000000000000000000, 10.00000000000000000, 1.000000000000000000 ) ) ;
#18428=DIRECTION ( 'NONE',  ( 1.000000000000000000, 0.000000000000000000, -0.000000000000000000 ) ) ;
#18434=CARTESIAN_POINT ( 'NONE',  ( -18.69064177244175795, 16.00000000000000000, 1.000000000000000000 ) ) ;
#18436=CARTESIAN_POINT ( 'NONE',  ( 14.31494360078803041, 10.00000000000000000, 0.000000000000000000 ) ) ;
#18444=VECTOR ( 'NONE', #13136, 1000.000000000000000 ) ;
#18453=EDGE_CURVE ( 'NONE', #19940, #19480, #3292, .T. ) ;
#18454=CARTESIAN_POINT ( 'NONE',  ( 30.80549002841696904, 5.431839045955454637, 1.000000000000000000 ) ) ;
#18457=FACE_OUTER_BOUND ( 'NONE', #149, .T. ) ;
#18469=LINE ( 'NONE', #10612, #15047 ) ;
#18470=ORIENTED_EDGE ( 'NONE', *, *, #14477, .F. ) ;
#18472=VECTOR ( 'NONE', #7661, 1000.000000000000000 ) ;
#18474=ORIENTED_EDGE ( 'NONE', *, *, #2619, .T. ) ;
#18477=CARTESIAN_POINT ( 'NONE',  ( 14.99999999999999645, 3.000000000000003553, 2.000000000000000000 ) ) ;
#18479=EDGE_CURVE ( 'NONE', #6038, #6263, #6545, .T. ) ;
#18483=PLANE ( 'NONE',  #17881 ) ;
#18486=DIRECTION ( 'NONE',  ( 1.000000000000000000, 0.000000000000000000, -0.000000000000000000 ) ) ;
#18500=ORIENTED_EDGE ( 'NONE', *, *, #7303, .F. ) ;
#18501=PRODUCT_CONTEXT ( 'NONE', #131, 'mechanical' ) ;
#18502=VERTEX_POINT ( 'NONE', #20576 ) ;
#18503=ORIENTED_EDGE ( 'NONE', *, *, #669, .F. ) ;
#18505=CARTESIAN_POINT ( 'NONE',  ( 0.000000000000000000, 10.00000000000000000, 1.000000000000000000 ) ) ;
#18506=EDGE_CURVE ( 'NONE', #19457, #18649, #1734, .T. ) ;
#18511=DIRECTION ( 'NONE',  ( 1.000000000000000000, 0.000000000000000000, 0.000000000000000000 ) ) ;
#18515=ORIENTED_EDGE ( 'NONE', *, *, #972, .T. ) ;
#18522=ORIENTED_EDGE ( 'NONE', *, *, #10983, .F. ) ;
#18525=LINE ( 'NONE', #2609, #7228 ) ;
#18527=FACE_OUTER_BOUND ( 'NONE', #6384, .T. ) ;
#18528=ORIENTED_EDGE ( 'NONE', *, *, #19410, .T. ) ;
#18537=DIRECTION ( 'NONE',  ( 1.000000000000000000, 0.000000000000000000, 0.000000000000000000 ) ) ;
#18542=ORIENTED_EDGE ( 'NONE', *, *, #20314, .T. ) ;
#18546=ORIENTED_EDGE ( 'NONE', *, *, #13595, .T. ) ;
#18552=CARTESIAN_POINT ( 'NONE',  ( -2.187849085826861550, 0.000000000000000000, 0.000000000000000000 ) ) ;
#18554=DIRECTION ( 'NONE',  ( 0.000000000000000000, 0.000000000000000000, -1.000000000000000000 ) ) ;
#18564=ORIENTED_EDGE ( 'NONE', *, *, #6673, .F. ) ;
#18566=DIRECTION ( 'NONE',  ( 1.000000000000000000, 0.000000000000000000, 0.000000000000000000 ) ) ;
#18568=VECTOR ( 'NONE', #19238, 1000.000000000000000 ) ;
#18571=EDGE_CURVE ( 'NONE', #14753, #11489, #256, .T. ) ;
#18602=DIRECTION ( 'NONE',  ( 1.000000000000000000, 0.000000000000000000, 0.000000000000000000 ) ) ;
#18605=CARTESIAN_POINT ( 'NONE',  ( -2.187849085826861550, 11.64110105645932691, 0.000000000000000000 ) ) ;
#18627=ORIENTED_EDGE ( 'NONE', *, *, #1472, .F. ) ;
#18645=PLANE ( 'NONE',  #5665 ) ;
#18647=AXIS2_PLACEMENT_3D ( 'NONE', #18830, #6989, #2172 ) ;
#18649=VERTEX_POINT ( 'NONE', #2442 ) ;
#18650=CARTESIAN_POINT ( 'NONE',  ( 12.25209451496117197, 10.00000000000000000, 1.000000000000000000 ) ) ;
#18658=PLANE ( 'NONE',  #10734 ) ;
#18679=VECTOR ( 'NONE', #14279, 1000.000000000000000 ) ;
#18680=VERTEX_POINT ( 'NONE', #11649 ) ;
#18681=DIRECTION ( 'NONE',  ( -1.000000000000000000, -1.156482317317871331E-15, 0.000000000000000000 ) ) ;
#18686=CARTESIAN_POINT ( 'NONE',  ( 2.687849085826861995, 0.000000000000000000, 1.000000000000000000 ) ) ;
#18689=VECTOR ( 'NONE', #9602, 1000.000000000000000 ) ;
#18691=CARTESIAN_POINT ( 'NONE',  ( 3.469446951953523943E-14, 10.00000000000009592, 1.000000000000000000 ) ) ;
#18701=ORIENTED_EDGE ( 'NONE', *, *, #14739, .F. ) ;
#18703=DIRECTION ( 'NONE',  ( 0.000000000000000000, 1.000000000000000000, -0.000000000000000000 ) ) ;
#18707=AXIS2_PLACEMENT_3D ( 'NONE', #4260, #9459, #7890 ) ;
#18709=CARTESIAN_POINT ( 'NONE',  ( -0.1250000000000001110, 0.000000000000000000, 0.000000000000000000 ) ) ;
#18710=LINE ( 'NONE', #18505, #12966 ) ;
#18713=CARTESIAN_POINT ( 'NONE',  ( -18.69064177244175795, 10.00000000000000000, 1.000000000000000000 ) ) ;
#18718=FACE_BOUND ( 'NONE', #9786, .T. ) ;
#18724=ORIENTED_EDGE ( 'NONE', *, *, #16428, .T. ) ;
#18729=ORIENTED_EDGE ( 'NONE', *, *, #16143, .F. ) ;
#18733=ORIENTED_EDGE ( 'NONE', *, *, #1281, .F. ) ;
#18740=VECTOR ( 'NONE', #12917, 1000.000000000000000 ) ;
#18741=AXIS2_PLACEMENT_3D ( 'NONE', #7478, #2548, #16979 ) ;
#18748=CARTESIAN_POINT ( 'NONE',  ( 27.44203811574919882, 16.00000000000000000, 1.000000000000000000 ) ) ;
#18752=VERTEX_POINT ( 'NONE', #5273 ) ;
#18758=AXIS2_PLACEMENT_3D ( 'NONE', #2958, #17701, #15712 ) ;
#18761=VECTOR ( 'NONE', #16480, 1000.000000000000000 ) ;
#18765=DIRECTION ( 'NONE',  ( 0.000000000000000000, 0.000000000000000000, -1.000000000000000000 ) ) ;
#18768=CARTESIAN_POINT ( 'NONE',  ( 21.25349085826861995, 11.64110105645932691, 0.000000000000000000 ) ) ;
#18769=DIRECTION ( 'NONE',  ( 1.000000000000000000, 0.000000000000000000, -0.000000000000000000 ) ) ;
#18773=ORIENTED_EDGE ( 'NONE', *, *, #6891, .T. ) ;
#18781=ORIENTED_EDGE ( 'NONE', *, *, #8231, .F. ) ;
#18782=ORIENTED_EDGE ( 'NONE', *, *, #4087, .F. ) ;
#18783=EDGE_CURVE ( 'NONE', #13004, #15521, #11639, .T. ) ;
#18784=DIRECTION ( 'NONE',  ( 0.000000000000000000, 0.000000000000000000, -1.000000000000000000 ) ) ;
#18785=ORIENTED_EDGE ( 'NONE', *, *, #5592, .T. ) ;
#18786=DIRECTION ( 'NONE',  ( 0.000000000000000000, -0.000000000000000000, 1.000000000000000000 ) ) ;
#18787=VECTOR ( 'NONE', #8002, 1000.000000000000000 ) ;
#18788=DIRECTION ( 'NONE',  ( 0.000000000000000000, 1.000000000000000000, 0.000000000000000000 ) ) ;
#18789=EDGE_LOOP ( 'NONE', ( #10928, #15548, #5835, #11034 ) ) ;
#18794=FACE_OUTER_BOUND ( 'NONE', #4161, .T. ) ;
#18798=CARTESIAN_POINT ( 'NONE',  ( -24.12918902992234393, 0.000000000000000000, 1.000000000000000000 ) ) ;
#18799=DIRECTION ( 'NONE',  ( -1.156482317317871133E-15, 1.000000000000000000, 0.000000000000000000 ) ) ;
#18809=FACE_OUTER_BOUND ( 'NONE', #6905, .T. ) ;
#18812=EDGE_CURVE ( 'NONE', #3441, #10513, #5483, .T. ) ;
#18813=ORIENTED_EDGE ( 'NONE', *, *, #10725, .F. ) ;
#18816=CARTESIAN_POINT ( 'NONE',  ( -29.71062960567704891, 11.64110105645932691, -1.734723475976807094E-15 ) ) ;
#18819=PLANE ( 'NONE',  #16998 ) ;
#18821=EDGE_CURVE ( 'NONE', #17687, #6665, #14794, .T. ) ;
#18830=CARTESIAN_POINT ( 'NONE',  ( -9.689245429134309973, 0.000000000000000000, 1.000000000000000000 ) ) ;
#18839=ORIENTED_EDGE ( 'NONE', *, *, #19803, .F. ) ;
#18842=AXIS2_PLACEMENT_3D ( 'NONE', #12871, #11411, #18784 ) ;
#18843=EDGE_CURVE ( 'NONE', #17840, #19958, #10502, .T. ) ;
#18851=PLANE ( 'NONE',  #12065 ) ;
#18853=AXIS2_PLACEMENT_3D ( 'NONE', #14989, #667, #5480 ) ;
#18864=PRODUCT ( 'Fixed Lower Stainless Steel Comb Blade', 'Fixed Lower Stainless Steel Comb Blade', '', ( #18501 ) ) ;
#18868=LINE ( 'NONE', #1289, #19235 ) ;
#18869=CARTESIAN_POINT ( 'NONE',  ( -15.87779268661489773, 16.00000000000000000, 1.000000000000000000 ) ) ;
#18876=PLANE ( 'NONE',  #20423 ) ;
#18881=DIRECTION ( 'NONE',  ( 0.000000000000000000, 1.000000000000000000, -0.000000000000000000 ) ) ;
#18882=EDGE_LOOP ( 'NONE', ( #18500, #20376, #13220, #2179 ) ) ;
#18883=ORIENTED_EDGE ( 'NONE', *, *, #10029, .T. ) ;
#18885=EDGE_CURVE ( 'NONE', #6147, #4809, #16974, .T. ) ;
#18886=ORIENTED_EDGE ( 'NONE', *, *, #4807, .T. ) ;
#18887=EDGE_CURVE ( 'NONE', #1368, #4053, #13933, .T. ) ;
#18889=VECTOR ( 'NONE', #440, 1000.000000000000000 ) ;
#18892=ORIENTED_EDGE ( 'NONE', *, *, #5174, .T. ) ;
#18898=CARTESIAN_POINT ( 'NONE',  ( 6.063547257480584207, 11.64110105645932691, 0.000000000000000000 ) ) ;
#18913=ORIENTED_EDGE ( 'NONE', *, *, #14537, .F. ) ;
#18917=LINE ( 'NONE', #19023, #10319 ) ;
#18924=FACE_OUTER_BOUND ( 'NONE', #1722, .T. ) ;
#18929=CARTESIAN_POINT ( 'NONE',  ( 0.000000000000000000, 10.00000000000000000, 1.000000000000000000 ) ) ;
#18938=DIRECTION ( 'NONE',  ( -0.000000000000000000, -0.000000000000000000, -1.000000000000000000 ) ) ;
#18942=CARTESIAN_POINT ( 'NONE',  ( 4.000698171653723101, 0.000000000000000000, 0.000000000000000000 ) ) ;
#18944=CARTESIAN_POINT ( 'NONE',  ( -15.00000000000000000, 0.000000000000000000, 2.000000000000000000 ) ) ;
#18945=VECTOR ( 'NONE', #5668, 1000.000000000000000 ) ;
#18949=ADVANCED_FACE ( 'NONE', ( #2762 ), #9140, .T. ) ;
#18958=EDGE_CURVE ( 'NONE', #13385, #2700, #636, .T. ) ;
#18960=VERTEX_POINT ( 'NONE', #10475 ) ;
#18961=ORIENTED_EDGE ( 'NONE', *, *, #20162, .F. ) ;
#18963=CIRCLE ( 'NONE', #9931, 10.00000000000000000 ) ;
#18976=ORIENTED_EDGE ( 'NONE', *, *, #184, .T. ) ;
#18978=PLANE ( 'NONE',  #6049 ) ;
#18987=ORIENTED_EDGE ( 'NONE', *, *, #18958, .F. ) ;
#18990=AXIS2_PLACEMENT_3D ( 'NONE', #12403, #5922, #4558 ) ;
#18998=DIRECTION ( 'NONE',  ( -1.000000000000000000, 0.000000000000000000, 0.000000000000000000 ) ) ;
#19004=AXIS2_PLACEMENT_3D ( 'NONE', #15660, #6470, #4783 ) ;
#19023=CARTESIAN_POINT ( 'NONE',  ( 15.00000000000000355, -5.999999999999996447, 2.000000000000000000 ) ) ;
#19026=LINE ( 'NONE', #4483, #14315 ) ;
#19035=DIRECTION ( 'NONE',  ( -1.000000000000000000, 0.000000000000000000, 0.000000000000000000 ) ) ;
#19037=AXIS2_PLACEMENT_3D ( 'NONE', #14260, #3094, #1421 ) ;
#19044=ORIENTED_EDGE ( 'NONE', *, *, #356, .F. ) ;
#19046=DIRECTION ( 'NONE',  ( 1.000000000000000000, 0.000000000000000000, 0.000000000000000000 ) ) ;
#19057=CARTESIAN_POINT ( 'NONE',  ( -0.1250000000000001110, 10.00000000000000000, 1.000000000000000000 ) ) ;
#19069=CIRCLE ( 'NONE', #19726, 10.00000000000000000 ) ;
#19071=DIRECTION ( 'NONE',  ( 0.000000000000000000, 0.000000000000000000, 1.000000000000000000 ) ) ;
#19073=DIRECTION ( 'NONE',  ( 0.000000000000000000, 1.000000000000000000, 0.000000000000000000 ) ) ;
#19074=PLANE ( 'NONE',  #1718 ) ;
#19077=EDGE_CURVE ( 'NONE', #1633, #16888, #10365, .T. ) ;
#19078=DIRECTION ( 'NONE',  ( -0.000000000000000000, -0.000000000000000000, -1.000000000000000000 ) ) ;
#19084=VECTOR ( 'NONE', #16674, 1000.000000000000000 ) ;
#19085=CARTESIAN_POINT ( 'NONE',  ( -11.75209451496117197, 0.000000000000000000, 0.000000000000000000 ) ) ;
#19086=VECTOR ( 'NONE', #10089, 1000.000000000000000 ) ;
#19096=EDGE_LOOP ( 'NONE', ( #3827, #15678, #5280, #16940 ) ) ;
#19097=CARTESIAN_POINT ( 'NONE',  ( 2.687849085826861995, 16.00000000000000000, 1.000000000000000000 ) ) ;
#19106=CARTESIAN_POINT ( 'NONE',  ( 0.000000000000000000, 10.00000000000000000, 1.000000000000000000 ) ) ;
#19107=CARTESIAN_POINT ( 'NONE',  ( 14.31494360078803041, 10.00000000000000000, 1.000000000000000000 ) ) ;
#19111=CARTESIAN_POINT ( 'NONE',  ( -9.689245429134309973, 10.00000000000000000, 1.000000000000000000 ) ) ;
#19122=VECTOR ( 'NONE', #13075, 1000.000000000000000 ) ;
#19124=ORIENTED_EDGE ( 'NONE', *, *, #19639, .T. ) ;
#19128=EDGE_CURVE ( 'NONE', #10227, #1283, #8588, .T. ) ;
#19150=VECTOR ( 'NONE', #658, 1000.000000000000000 ) ;
#19151=ADVANCED_FACE ( 'NONE', ( #13593 ), #7134, .T. ) ;
#19152=DIRECTION ( 'NONE',  ( 0.000000000000000000, 1.000000000000000000, -0.000000000000000000 ) ) ;
#19154=EDGE_LOOP ( 'NONE', ( #2265, #18785, #12606, #3587 ) ) ;
#19157=EDGE_CURVE ( 'NONE', #11568, #3392, #9208, .T. ) ;
#19173=FACE_OUTER_BOUND ( 'NONE', #19096, .T. ) ;
#19174=ORIENTED_EDGE ( 'NONE', *, *, #1281, .T. ) ;
#19175=EDGE_LOOP ( 'NONE', ( #10805, #2851, #104, #9280 ) ) ;
#19178=DIRECTION ( 'NONE',  ( 1.000000000000000000, 0.000000000000000000, -0.000000000000000000 ) ) ;
#19185=CARTESIAN_POINT ( 'NONE',  ( 5.381197846483058989, -14.00000000000000000, 1.000000000000000000 ) ) ;
#19190=LINE ( 'NONE', #14353, #2361 ) ;
#19194=ORIENTED_EDGE ( 'NONE', *, *, #3855, .F. ) ;
#19199=ORIENTED_EDGE ( 'NONE', *, *, #4292, .T. ) ;
#19200=DIRECTION ( 'NONE',  ( -1.000000000000000000, -1.734723475976787570E-15, 0.000000000000000000 ) ) ;
#19201=LINE ( 'NONE', #7894, #9228 ) ;
#19202=DIRECTION ( 'NONE',  ( 0.000000000000000000, -1.000000000000000000, 0.000000000000000000 ) ) ;
#19203=CARTESIAN_POINT ( 'NONE',  ( -14.56494360078803396, 10.00000000000000000, 1.000000000000000000 ) ) ;
#19211=CARTESIAN_POINT ( 'NONE',  ( -0.1250000000000001110, 11.64110105645932691, 0.000000000000000000 ) ) ;
#19220=CARTESIAN_POINT ( 'NONE',  ( -26.94203811574920593, 0.000000000000000000, 1.000000000000000000 ) ) ;
#19224=VERTEX_POINT ( 'NONE', #7324 ) ;
#19225=DIRECTION ( 'NONE',  ( 0.000000000000000000, 1.000000000000000000, 0.000000000000000000 ) ) ;
#19231=VECTOR ( 'NONE', #3570, 1000.000000000000000 ) ;
#19235=VECTOR ( 'NONE', #6106, 1000.000000000000000 ) ;
#19236=DIRECTION ( 'NONE',  ( -0.000000000000000000, -0.000000000000000000, -1.000000000000000000 ) ) ;
#19238=DIRECTION ( 'NONE',  ( -0.000000000000000000, -0.000000000000000000, -1.000000000000000000 ) ) ;
#19240=EDGE_CURVE ( 'NONE', #3754, #346, #11985, .T. ) ;
#19247=LINE ( 'NONE', #1969, #15000 ) ;
#19252=EDGE_LOOP ( 'NONE', ( #11995, #3722, #12362, #13032, #655, #6307, #14294, #10863, #6046, #1249, #11182, #3973, #12213, #17849, #8710, #16641, #14697, #11156, #18503, #9811, #6372, #15284, #15059, #8933, #20569, #10956, #8875, #1723, #17087, #14181, #5253, #17631, #1365, #17283, #13029, #5572, #19622, #20323, #19627, #4109, #2053, #19890, #1598, #13225, #19459, #12918, #7937, #12610, #17995, #14593, #12529, #16453, #6459, #13365, #6074, #10694, #18729, #4208, #5473, #12516, #3691, #9482, #13898, #4646, #4396, #2348, #1342, #20302, #13512, #10415, #1810, #10779, #5800, #16665, #15778, #9501, #3013, #245, #18813, #5087, #9896, #15852, #2634, #17824, #9294, #12849, #13852, #16760, #6111, #1500, #6762, #14257, #9796, #14678, #9384, #3306, #17342, #5423, #17069, #3131, #18340, #11915, #14274, #11692, #7100, #19618, #5134, #2325, #12026, #20687, #4241, #3303, #12286, #991, #11796, #13247, #4723, #18782, #15733, #629, #11092, #9225, #1295, #1156 ) ) ;
#19253=EDGE_CURVE ( 'NONE', #19324, #4668, #4181, .T. ) ;
#19255=LINE ( 'NONE', #6588, #5250 ) ;
#19265=DIRECTION ( 'NONE',  ( 1.000000000000000000, 0.000000000000000000, 0.000000000000000000 ) ) ;
#19274=DIRECTION ( 'NONE',  ( -1.000000000000000000, 0.000000000000000000, 0.000000000000000000 ) ) ;
#19276=EDGE_LOOP ( 'NONE', ( #12340, #17293, #19485, #1585 ) ) ;
#19279=DIRECTION ( 'NONE',  ( 0.000000000000000000, 0.000000000000000000, -1.000000000000000000 ) ) ;
#19283=DIRECTION ( 'NONE',  ( 0.000000000000000000, -1.000000000000000000, 0.000000000000000000 ) ) ;
#19284=DIRECTION ( 'NONE',  ( 1.156482317317871971E-16, -1.000000000000000000, 0.000000000000000000 ) ) ;
#19296=EDGE_LOOP ( 'NONE', ( #20535, #8438, #13126, #19577 ) ) ;
#19301=ORIENTED_EDGE ( 'NONE', *, *, #10013, .T. ) ;
#19302=CARTESIAN_POINT ( 'NONE',  ( 27.00000000000000000, 0.000000000000000000, 1.000000000000000000 ) ) ;
#19304=DIRECTION ( 'NONE',  ( 0.000000000000000000, -0.000000000000000000, 1.000000000000000000 ) ) ;
#19305=ORIENTED_EDGE ( 'NONE', *, *, #7980, .T. ) ;
#19314=PLANE ( 'NONE',  #14018 ) ;
#19318=ORIENTED_EDGE ( 'NONE', *, *, #3496, .T. ) ;
#19320=LINE ( 'NONE', #4977, #11704 ) ;
#19323=DIRECTION ( 'NONE',  ( 1.000000000000000000, 0.000000000000000000, 0.000000000000000000 ) ) ;
#19324=VERTEX_POINT ( 'NONE', #15057 ) ;
#19326=VECTOR ( 'NONE', #4158, 1000.000000000000000 ) ;
#19327=ORIENTED_EDGE ( 'NONE', *, *, #2619, .F. ) ;
#19329=DIRECTION ( 'NONE',  ( -1.000000000000000000, 0.000000000000000000, 0.000000000000000000 ) ) ;
#19341=VERTEX_POINT ( 'NONE', #15260 ) ;
#19345=ORIENTED_EDGE ( 'NONE', *, *, #20443, .F. ) ;
#19346=DIRECTION ( 'NONE',  ( 0.000000000000000000, 0.000000000000000000, -1.000000000000000000 ) ) ;
#19352=DIRECTION ( 'NONE',  ( 6.938893903907228378E-16, -1.000000000000000000, 0.000000000000000000 ) ) ;
#19353=AXIS2_PLACEMENT_3D ( 'NONE', #4165, #20282, #12313 ) ;
#19354=VERTEX_POINT ( 'NONE', #3869 ) ;
#19358=LINE ( 'NONE', #14313, #14134 ) ;
#19361=DIRECTION ( 'NONE',  ( -1.000000000000000000, 0.000000000000000000, 0.000000000000000000 ) ) ;
#19363=AXIS2_PLACEMENT_3D ( 'NONE', #17926, #19515, #6749 ) ;
#19376=LINE ( 'NONE', #16125, #4476 ) ;
#19385=LINE ( 'NONE', #20570, #6858 ) ;
#19387=VECTOR ( 'NONE', #6799, 1000.000000000000000 ) ;
#19397=LINE ( 'NONE', #4634, #3369 ) ;
#19401=ORIENTED_EDGE ( 'NONE', *, *, #1493, .T. ) ;
#19404=FACE_OUTER_BOUND ( 'NONE', #5523, .T. ) ;
#19406=VECTOR ( 'NONE', #1733, 1000.000000000000000 ) ;
#19407=VERTEX_POINT ( 'NONE', #20095 ) ;
#19408=DIRECTION ( 'NONE',  ( -0.000000000000000000, -0.000000000000000000, -1.000000000000000000 ) ) ;
#19410=EDGE_CURVE ( 'NONE', #12443, #11466, #4495, .T. ) ;
#19411=DIRECTION ( 'NONE',  ( -0.000000000000000000, -1.000000000000000000, -0.000000000000000000 ) ) ;
#19417=AXIS2_PLACEMENT_3D ( 'NONE', #14773, #2137, #2233 ) ;
#19420=CARTESIAN_POINT ( 'NONE',  ( -11.75209451496117197, 11.64110105645932691, 0.000000000000000000 ) ) ;
#19434=ORIENTED_EDGE ( 'NONE', *, *, #1207, .F. ) ;
#19435=FACE_OUTER_BOUND ( 'NONE', #16732, .T. ) ;
#19437=VECTOR ( 'NONE', #8909, 1000.000000000000000 ) ;
#19439=CARTESIAN_POINT ( 'NONE',  ( -11.75209451496117197, 0.000000000000000000, 1.000000000000000000 ) ) ;
#19445=LINE ( 'NONE', #17958, #8874 ) ;
#19447=VECTOR ( 'NONE', #93, 1000.000000000000000 ) ;
#19452=ORIENTED_EDGE ( 'NONE', *, *, #9276, .T. ) ;
#19457=VERTEX_POINT ( 'NONE', #3032 ) ;
#19459=ORIENTED_EDGE ( 'NONE', *, *, #8511, .F. ) ;
#19465=DIRECTION ( 'NONE',  ( 1.000000000000000000, 0.000000000000000000, 0.000000000000000000 ) ) ;
#19471=AXIS2_PLACEMENT_3D ( 'NONE', #1792, #15523, #13848 ) ;
#19474=DIRECTION ( 'NONE',  ( 0.000000000000000000, 1.000000000000000000, 0.000000000000000000 ) ) ;
#19480=VERTEX_POINT ( 'NONE', #7531 ) ;
#19484=DIRECTION ( 'NONE',  ( 0.4999999999999949485, -0.8660254037844415942, 0.000000000000000000 ) ) ;
#19485=ORIENTED_EDGE ( 'NONE', *, *, #12681, .F. ) ;
#19487=EDGE_CURVE ( 'NONE', #9004, #3619, #15781, .T. ) ;
#19497=CARTESIAN_POINT ( 'NONE',  ( -1.437849085826860884, 0.000000000000000000, 1.000000000000000000 ) ) ;
#19501=LINE ( 'NONE', #5154, #368 ) ;
#19509=LINE ( 'NONE', #14675, #319 ) ;
#19510=ORIENTED_EDGE ( 'NONE', *, *, #6856, .T. ) ;
#19511=ORIENTED_EDGE ( 'NONE', *, *, #11563, .F. ) ;
#19515=DIRECTION ( 'NONE',  ( 1.000000000000000000, 0.000000000000000000, -0.000000000000000000 ) ) ;
#19523=EDGE_LOOP ( 'NONE', ( #9737, #10028, #5861, #14622 ) ) ;
#19528=ORIENTED_EDGE ( 'NONE', *, *, #9473, .F. ) ;
#19532=ORIENTED_EDGE ( 'NONE', *, *, #13362, .T. ) ;
#19535=ORIENTED_EDGE ( 'NONE', *, *, #5330, .T. ) ;
#19536=DIRECTION ( 'NONE',  ( 0.000000000000000000, -0.000000000000000000, 1.000000000000000000 ) ) ;
#19537=ORIENTED_EDGE ( 'NONE', *, *, #13497, .T. ) ;
#19558=DIRECTION ( 'NONE',  ( 1.000000000000000000, 0.000000000000000000, 0.000000000000000000 ) ) ;
#19572=CARTESIAN_POINT ( 'NONE',  ( -13.81494360078803396, 0.000000000000000000, 1.000000000000000000 ) ) ;
#19573=DIRECTION ( 'NONE',  ( -0.000000000000000000, -0.000000000000000000, -1.000000000000000000 ) ) ;
#19577=ORIENTED_EDGE ( 'NONE', *, *, #18571, .T. ) ;
#19580=ORIENTED_EDGE ( 'NONE', *, *, #5958, .F. ) ;
#19582=DIRECTION ( 'NONE',  ( 0.000000000000000000, 1.000000000000000000, -0.000000000000000000 ) ) ;
#19603=CARTESIAN_POINT ( 'NONE',  ( 19.19064177244175440, 0.000000000000000000, 1.000000000000000000 ) ) ;
#19606=CARTESIAN_POINT ( 'NONE',  ( -15.87779268661489773, 10.00000000000000000, 1.000000000000000000 ) ) ;
#19608=LINE ( 'NONE', #5263, #20676 ) ;
#19612=CARTESIAN_POINT ( 'NONE',  ( -0.000000000000000000, 10.00000000000000000, 0.000000000000000000 ) ) ;
#19614=CARTESIAN_POINT ( 'NONE',  ( -11.75209451496117197, 11.64110105645932691, 10.00000000000000000 ) ) ;
#19618=ORIENTED_EDGE ( 'NONE', *, *, #14349, .F. ) ;
#19622=ORIENTED_EDGE ( 'NONE', *, *, #949, .F. ) ;
#19626=EDGE_CURVE ( 'NONE', #9770, #10279, #17968, .T. ) ;
#19627=ORIENTED_EDGE ( 'NONE', *, *, #4292, .F. ) ;
#19637=DIRECTION ( 'NONE',  ( 1.000000000000000000, 0.000000000000000000, 0.000000000000000000 ) ) ;
#19639=EDGE_CURVE ( 'NONE', #8046, #3441, #196, .T. ) ;
#19650=DIRECTION ( 'NONE',  ( 0.000000000000000000, 1.000000000000000000, -0.000000000000000000 ) ) ;
#19652=ORIENTED_EDGE ( 'NONE', *, *, #12135, .F. ) ;
#19656=DIRECTION ( 'NONE',  ( -1.000000000000000000, 0.000000000000000000, 0.000000000000000000 ) ) ;
#19658=VECTOR ( 'NONE', #7287, 1000.000000000000000 ) ;
#19662=SHAPE_REPRESENTATION ( 'Fixed Lower Stainless Steel Comb Blade', ( #18039 ), #5348 ) ;
#19669=LINE ( 'NONE', #5334, #17764 ) ;
#19673=VECTOR ( 'NONE', #11347, 1000.000000000000000 ) ;
#19674=EDGE_LOOP ( 'NONE', ( #1389, #15592, #2774, #7172 ) ) ;
#19678=PLANE ( 'NONE',  #4016 ) ;
#19679=VERTEX_POINT ( 'NONE', #405 ) ;
#19685=VECTOR ( 'NONE', #466, 1000.000000000000000 ) ;
#19689=CARTESIAN_POINT ( 'NONE',  ( -9.689245429134309973, 10.00000000000000000, 0.000000000000000000 ) ) ;
#19692=LINE ( 'NONE', #2738, #2057 ) ;
#19695=VECTOR ( 'NONE', #10103, 1000.000000000000000 ) ;
#19699=ORIENTED_EDGE ( 'NONE', *, *, #197, .T. ) ;
#19704=VERTEX_POINT ( 'NONE', #4801 ) ;
#19705=EDGE_CURVE ( 'NONE', #962, #2639, #20712, .T. ) ;
#19713=CYLINDRICAL_SURFACE ( 'NONE', #14982, 10.00000000000000000 ) ;
#19726=AXIS2_PLACEMENT_3D ( 'NONE', #12876, #1699, #13186 ) ;
#19733=DIRECTION ( 'NONE',  ( 0.000000000000000000, 1.000000000000000000, -0.000000000000000000 ) ) ;
#19736=CARTESIAN_POINT ( 'NONE',  ( 9.000000000000000000, -9.999999999999991118, 2.000000000000000000 ) ) ;
#19740=ORIENTED_EDGE ( 'NONE', *, *, #18198, .T. ) ;
#19745=CARTESIAN_POINT ( 'NONE',  ( -20.75349085826862350, 0.000000000000000000, 1.000000000000000000 ) ) ;
#19751=LINE ( 'NONE', #13454, #13221 ) ;
#19762=CIRCLE ( 'NONE', #13395, 10.00000000000000000 ) ;
#19763=EDGE_CURVE ( 'NONE', #20538, #17687, #19247, .T. ) ;
#19767=DIRECTION ( 'NONE',  ( 0.000000000000000000, 0.000000000000000000, -1.000000000000000000 ) ) ;
#19768=ORIENTED_EDGE ( 'NONE', *, *, #13976, .T. ) ;
#19791=DIRECTION ( 'NONE',  ( 1.000000000000000000, 0.000000000000000000, 0.000000000000000000 ) ) ;
#19800=CARTESIAN_POINT ( 'NONE',  ( 19.19064177244175440, 10.00000000000000000, 1.000000000000000000 ) ) ;
#19803=EDGE_CURVE ( 'NONE', #10907, #11591, #604, .T. ) ;
#19807=DIRECTION ( 'NONE',  ( 1.000000000000000000, 0.000000000000000000, 0.000000000000000000 ) ) ;
#19809=AXIS2_PLACEMENT_3D ( 'NONE', #5092, #19225, #16278 ) ;
#19814=ORIENTED_EDGE ( 'NONE', *, *, #13573, .F. ) ;
#19817=CARTESIAN_POINT ( 'NONE',  ( 17.12779268661489596, 11.64110105645932691, 10.00000000000000000 ) ) ;
#19822=CARTESIAN_POINT ( 'NONE',  ( 10.18924542913430820, 0.000000000000000000, 1.000000000000000000 ) ) ;
#19823=DIRECTION ( 'NONE',  ( 0.4999999999999947820, 0.8660254037844417052, -0.000000000000000000 ) ) ;
#19824=DIRECTION ( 'NONE',  ( 0.000000000000000000, -1.000000000000000000, 0.000000000000000000 ) ) ;
#19826=DIRECTION ( 'NONE',  ( 1.000000000000000000, 0.000000000000000000, 0.000000000000000000 ) ) ;
#19828=ADVANCED_FACE ( 'NONE', ( #913 ), #16811, .T. ) ;
#19836=AXIS2_PLACEMENT_3D ( 'NONE', #17875, #6583, #14524 ) ;
#19840=LINE ( 'NONE', #12078, #19084 ) ;
#19841=ORIENTED_EDGE ( 'NONE', *, *, #9135, .T. ) ;
#19843=CARTESIAN_POINT ( 'NONE',  ( 19.19064177244175440, 0.000000000000000000, 1.000000000000000000 ) ) ;
#19846=VECTOR ( 'NONE', #5811, 1000.000000000000000 ) ;
#19848=ORIENTED_EDGE ( 'NONE', *, *, #10520, .F. ) ;
#19856=CARTESIAN_POINT ( 'NONE',  ( -0.1250000000000001110, 10.00000000000000000, 1.000000000000000000 ) ) ;
#19858=DIRECTION ( 'NONE',  ( -0.000000000000000000, -0.000000000000000000, -1.000000000000000000 ) ) ;
#19873=CARTESIAN_POINT ( 'NONE',  ( -13.81494360078803396, 11.64110105645932691, 0.000000000000000000 ) ) ;
#19876=DIRECTION ( 'NONE',  ( 1.000000000000000000, 0.000000000000000000, 0.000000000000000000 ) ) ;
#19879=LINE ( 'NONE', #7423, #5684 ) ;
#19888=DIRECTION ( 'NONE',  ( 1.000000000000000000, 0.000000000000000000, -0.000000000000000000 ) ) ;
#19889=ORIENTED_EDGE ( 'NONE', *, *, #8750, .F. ) ;
#19890=ORIENTED_EDGE ( 'NONE', *, *, #4163, .F. ) ;
#19903=LINE ( 'NONE', #10372, #7722 ) ;
#19914=ORIENTED_EDGE ( 'NONE', *, *, #16608, .T. ) ;
#19919=EDGE_CURVE ( 'NONE', #10855, #11555, #5309, .T. ) ;
#19920=VERTEX_POINT ( 'NONE', #10226 ) ;
#19923=CARTESIAN_POINT ( 'NONE',  ( 20.50349085826861995, 10.00000000000000000, 1.000000000000000000 ) ) ;
#19924=CARTESIAN_POINT ( 'NONE',  ( 30.00000000000000000, 0.000000000000000000, 0.000000000000000000 ) ) ;
#19926=CARTESIAN_POINT ( 'NONE',  ( 13.00209451496117374, 11.64110105645932691, 10.00000000000000000 ) ) ;
#19927=CARTESIAN_POINT ( 'NONE',  ( 18.44064177244175440, 0.000000000000000000, 1.000000000000000000 ) ) ;
#19932=EDGE_LOOP ( 'NONE', ( #4056, #4347, #4744, #15732 ) ) ;
#19934=CARTESIAN_POINT ( 'NONE',  ( 4.000698171653723101, 10.00000000000000000, 1.000000000000000000 ) ) ;
#19940=VERTEX_POINT ( 'NONE', #7300 ) ;
#19943=DIRECTION ( 'NONE',  ( -0.000000000000000000, -0.000000000000000000, -1.000000000000000000 ) ) ;
#19944=ORIENTED_EDGE ( 'NONE', *, *, #5995, .F. ) ;
#19947=DIRECTION ( 'NONE',  ( -0.000000000000000000, 0.000000000000000000, -1.000000000000000000 ) ) ;
#19949=CARTESIAN_POINT ( 'NONE',  ( 0.000000000000000000, 0.000000000000000000, 1.000000000000000000 ) ) ;
#19955=DIRECTION ( 'NONE',  ( 1.000000000000000000, 0.000000000000000000, 0.000000000000000000 ) ) ;
#19958=VERTEX_POINT ( 'NONE', #503 ) ;
#19961=EDGE_LOOP ( 'NONE', ( #8560, #5310, #20462, #6291 ) ) ;
#19964=VERTEX_POINT ( 'NONE', #5625 ) ;
#19966=VECTOR ( 'NONE', #12636, 1000.000000000000000 ) ;
#19968=EDGE_CURVE ( 'NONE', #11652, #17187, #9990, .T. ) ;
#19971=CARTESIAN_POINT ( 'NONE',  ( 10.18924542913430820, 10.00000000000000000, 1.000000000000000000 ) ) ;
#19974=FACE_OUTER_BOUND ( 'NONE', #17801, .T. ) ;
#19976=CARTESIAN_POINT ( 'NONE',  ( 13.00209451496117374, 10.00000000000000000, 1.000000000000000000 ) ) ;
#19980=EDGE_LOOP ( 'NONE', ( #2427, #9465, #20492, #271 ) ) ;
#19991=ADVANCED_FACE ( 'NONE', ( #6883 ), #2173, .T. ) ;
#19996=DIRECTION ( 'NONE',  ( 1.000000000000000000, -0.000000000000000000, 0.000000000000000000 ) ) ;
#19998=PLANE ( 'NONE',  #15194 ) ;
#20003=VECTOR ( 'NONE', #13670, 1000.000000000000000 ) ;
#20020=LINE ( 'NONE', #5683, #12779 ) ;
#20026=CARTESIAN_POINT ( 'NONE',  ( 8.126396343307449754, 0.000000000000000000, 0.000000000000000000 ) ) ;
#20029=CARTESIAN_POINT ( 'NONE',  ( 0.000000000000000000, 16.00000000000000000, 1.000000000000000000 ) ) ;
#20035=VERTEX_POINT ( 'NONE', #12206 ) ;
#20040=CIRCLE ( 'NONE', #14677, 10.00000000000000000 ) ;
#20041=ORIENTED_EDGE ( 'NONE', *, *, #11501, .T. ) ;
#20048=EDGE_CURVE ( 'NONE', #6320, #3666, #2584, .T. ) ;
#20050=AXIS2_PLACEMENT_3D ( 'NONE', #6517, #16510, #16026 ) ;
#20051=VERTEX_POINT ( 'NONE', #16046 ) ;
#20052=FACE_OUTER_BOUND ( 'NONE', #6715, .T. ) ;
#20061=LINE ( 'NONE', #11577, #10634 ) ;
#20071=CARTESIAN_POINT ( 'NONE',  ( -26.19203811574920593, 10.00000000000000000, 1.000000000000000000 ) ) ;
#20073=ORIENTED_EDGE ( 'NONE', *, *, #20048, .F. ) ;
#20075=VECTOR ( 'NONE', #7597, 1000.000000000000000 ) ;
#20077=CARTESIAN_POINT ( 'NONE',  ( -9.000000000000000000, -9.999999999999992895, 2.000000000000000000 ) ) ;
#20078=CARTESIAN_POINT ( 'NONE',  ( 0.000000000000000000, 0.000000000000000000, 1.000000000000000000 ) ) ;
#20085=VECTOR ( 'NONE', #18566, 1000.000000000000000 ) ;
#20087=VECTOR ( 'NONE', #9453, 1000.000000000000000 ) ;
#20089=AXIS2_PLACEMENT_3D ( 'NONE', #20310, #7342, #15177 ) ;
#20095=CARTESIAN_POINT ( 'NONE',  ( -26.94203811574920593, 10.00000000000000000, 1.000000000000000000 ) ) ;
#20097=ORIENTED_EDGE ( 'NONE', *, *, #2132, .F. ) ;
#20101=VERTEX_POINT ( 'NONE', #16911 ) ;
#20105=VECTOR ( 'NONE', #470, 1000.000000000000000 ) ;
#20111=DIRECTION ( 'NONE',  ( 1.000000000000000000, 0.000000000000000000, 0.000000000000000000 ) ) ;
#20116=VECTOR ( 'NONE', #11708, 1000.000000000000000 ) ;
#20119=VERTEX_POINT ( 'NONE', #20177 ) ;
#20120=ADVANCED_FACE ( 'NONE', ( #1024 ), #6431, .T. ) ;
#20126=ORIENTED_EDGE ( 'NONE', *, *, #2061, .F. ) ;
#20127=CARTESIAN_POINT ( 'NONE',  ( 0.000000000000000000, 16.00000000000000000, 1.000000000000000000 ) ) ;
#20128=CARTESIAN_POINT ( 'NONE',  ( -5.381197846483055436, -6.000000000000000000, 2.000000000000000000 ) ) ;
#20132=DIRECTION ( 'NONE',  ( -0.1736481776669293042, 0.9848077530122082424, 0.000000000000000000 ) ) ;
#20134=LINE ( 'NONE', #15199, #17167 ) ;
#20151=CARTESIAN_POINT ( 'NONE',  ( 12.25209451496117197, 0.000000000000000000, 1.000000000000000000 ) ) ;
#20152=ORIENTED_EDGE ( 'NONE', *, *, #1736, .F. ) ;
#20157=DIRECTION ( 'NONE',  ( 0.000000000000000000, 0.000000000000000000, -1.000000000000000000 ) ) ;
#20158=CARTESIAN_POINT ( 'NONE',  ( -0.000000000000000000, 11.64110105645932691, 0.000000000000000000 ) ) ;
#20161=AXIS2_PLACEMENT_3D ( 'NONE', #18000, #17899, #16232 ) ;
#20162=EDGE_CURVE ( 'NONE', #6206, #2900, #12795, .T. ) ;
#20165=CARTESIAN_POINT ( 'NONE',  ( 0.6250000000000005551, 0.000000000000000000, 1.000000000000000000 ) ) ;
#20167=CARTESIAN_POINT ( 'NONE',  ( -5.563547257480587760, 11.64110105645932691, 0.000000000000000000 ) ) ;
#20169=FACE_OUTER_BOUND ( 'NONE', #7274, .T. ) ;
#20177=CARTESIAN_POINT ( 'NONE',  ( 18.44064177244175440, 11.64110105645932691, 0.000000000000000000 ) ) ;
#20178=VECTOR ( 'NONE', #19465, 1000.000000000000000 ) ;
#20179=ORIENTED_EDGE ( 'NONE', *, *, #10396, .T. ) ;
#20182=EDGE_CURVE ( 'NONE', #9838, #7608, #19509, .T. ) ;
#20184=ORIENTED_EDGE ( 'NONE', *, *, #13519, .T. ) ;
#20185=CARTESIAN_POINT ( 'NONE',  ( -0.1250000000000001110, 0.000000000000000000, 1.000000000000000000 ) ) ;
#20186=DIRECTION ( 'NONE',  ( 0.000000000000000000, 1.000000000000000000, -0.000000000000000000 ) ) ;
#20199=DIRECTION ( 'NONE',  ( 1.000000000000000000, 0.000000000000000000, 0.000000000000000000 ) ) ;
#20200=ORIENTED_EDGE ( 'NONE', *, *, #11067, .F. ) ;
#20203=CARTESIAN_POINT ( 'NONE',  ( 0.000000000000000000, 16.00000000000000000, 1.000000000000000000 ) ) ;
#20212=DIRECTION ( 'NONE',  ( -0.000000000000000000, -0.000000000000000000, -1.000000000000000000 ) ) ;
#20225=CARTESIAN_POINT ( 'NONE',  ( -29.71062960567704891, 11.64110105645932691, -1.734723475976807094E-15 ) ) ;
#20228=AXIS2_PLACEMENT_3D ( 'NONE', #18477, #18681, #4348 ) ;
#20235=EDGE_CURVE ( 'NONE', #14721, #12182, #20040, .T. ) ;
#20236=CARTESIAN_POINT ( 'NONE',  ( 0.000000000000000000, 10.00000000000000000, 1.000000000000000000 ) ) ;
#20253=ADVANCED_FACE ( 'NONE', ( #19404 ), #9768, .T. ) ;
#20256=DIRECTION ( 'NONE',  ( 1.000000000000000000, -0.000000000000000000, 0.000000000000000000 ) ) ;
#20263=LINE ( 'NONE', #1325, #2295 ) ;
#20264=LINE ( 'NONE', #18691, #20075 ) ;
#20268=ADVANCED_FACE ( 'NONE', ( #5365 ), #5062, .T. ) ;
#20275=VECTOR ( 'NONE', #15371, 1000.000000000000000 ) ;
#20276=DIRECTION ( 'NONE',  ( 0.000000000000000000, -1.000000000000000000, 0.000000000000000000 ) ) ;
#20279=ADVANCED_FACE ( 'NONE', ( #2224 ), #9866, .T. ) ;
#20281=ORIENTED_EDGE ( 'NONE', *, *, #16428, .F. ) ;
#20282=DIRECTION ( 'NONE',  ( 1.000000000000000000, 0.000000000000000000, -0.000000000000000000 ) ) ;
#20283=CYLINDRICAL_SURFACE ( 'NONE', #280, 10.00000000000000000 ) ;
#20287=CARTESIAN_POINT ( 'NONE',  ( -10.38119784648305632, -14.00000000000000000, 1.000000000000000000 ) ) ;
#20302=ORIENTED_EDGE ( 'NONE', *, *, #11779, .F. ) ;
#20310=CARTESIAN_POINT ( 'NONE',  ( 17.12779268661489596, 0.000000000000000000, 1.000000000000000000 ) ) ;
#20314=EDGE_CURVE ( 'NONE', #10279, #2639, #11539, .T. ) ;
#20323=ORIENTED_EDGE ( 'NONE', *, *, #1099, .F. ) ;
#20325=ORIENTED_EDGE ( 'NONE', *, *, #7932, .T. ) ;
#20334=DIRECTION ( 'NONE',  ( -0.000000000000000000, -0.000000000000000000, -1.000000000000000000 ) ) ;
#20344=ORIENTED_EDGE ( 'NONE', *, *, #5170, .T. ) ;
#20350=DIRECTION ( 'NONE',  ( 1.000000000000000000, 0.000000000000000000, 0.000000000000000000 ) ) ;
#20353=FACE_OUTER_BOUND ( 'NONE', #5628, .T. ) ;
#20356=VECTOR ( 'NONE', #18602, 1000.000000000000000 ) ;
#20360=DIRECTION ( 'NONE',  ( -1.000000000000000000, 0.000000000000000000, 0.000000000000000000 ) ) ;
#20367=VECTOR ( 'NONE', #20199, 1000.000000000000000 ) ;
#20368=CARTESIAN_POINT ( 'NONE',  ( -4.250698171653726654, 0.000000000000000000, 0.000000000000000000 ) ) ;
#20369=LINE ( 'NONE', #17423, #12724 ) ;
#20374=EDGE_CURVE ( 'NONE', #9634, #4496, #18135, .T. ) ;
#20376=ORIENTED_EDGE ( 'NONE', *, *, #9359, .T. ) ;
#20378=FACE_OUTER_BOUND ( 'NONE', #16427, .T. ) ;
#20383=EDGE_CURVE ( 'NONE', #19224, #13004, #15394, .T. ) ;
#20384=CIRCLE ( 'NONE', #13002, 10.00000000000000000 ) ;
#20387=VECTOR ( 'NONE', #17839, 1000.000000000000000 ) ;
#20388=ORIENTED_EDGE ( 'NONE', *, *, #1652, .T. ) ;
#20389=DIRECTION ( 'NONE',  ( 0.000000000000000000, 0.000000000000000000, 1.000000000000000000 ) ) ;
#20397=CARTESIAN_POINT ( 'NONE',  ( -9.689245429134309973, 10.00000000000000000, 1.000000000000000000 ) ) ;
#20399=ADVANCED_FACE ( 'NONE', ( #766 ), #18645, .T. ) ;
#20402=DIRECTION ( 'NONE',  ( 1.000000000000000000, 0.000000000000000000, -0.000000000000000000 ) ) ;
#20405=CIRCLE ( 'NONE', #14362, 10.00000000000000000 ) ;
#20408=VERTEX_POINT ( 'NONE', #16759 ) ;
#20409=ORIENTED_EDGE ( 'NONE', *, *, #7758, .F. ) ;
#20414=CARTESIAN_POINT ( 'NONE',  ( -0.000000000000000000, 11.64110105645932691, 0.000000000000000000 ) ) ;
#20416=EDGE_CURVE ( 'NONE', #8358, #13991, #12153, .T. ) ;
#20418=DIRECTION ( 'NONE',  ( -1.000000000000000000, -5.782411586589356653E-16, 0.000000000000000000 ) ) ;
#20423=AXIS2_PLACEMENT_3D ( 'NONE', #15614, #7787, #8935 ) ;
#20424=AXIS2_PLACEMENT_3D ( 'NONE', #6615, #9752, #15815 ) ;
#20437=AXIS2_PLACEMENT_3D ( 'NONE', #16418, #14538, #9733 ) ;
#20438=CYLINDRICAL_SURFACE ( 'NONE', #8335, 10.00000000000000000 ) ;
#20443=EDGE_CURVE ( 'NONE', #12487, #9838, #15690, .T. ) ;
#20447=DIRECTION ( 'NONE',  ( -0.000000000000000000, 0.000000000000000000, 1.000000000000000000 ) ) ;
#20451=VECTOR ( 'NONE', #8682, 1000.000000000000000 ) ;
#20454=VERTEX_POINT ( 'NONE', #7353 ) ;
#20459=EDGE_LOOP ( 'NONE', ( #17943, #18913, #4369, #17873 ) ) ;
#20462=ORIENTED_EDGE ( 'NONE', *, *, #27, .T. ) ;
#20463=VERTEX_POINT ( 'NONE', #10589 ) ;
#20467=AXIS2_PLACEMENT_3D ( 'NONE', #3283, #6321, #7893 ) ;
#20476=DIRECTION ( 'NONE',  ( 1.000000000000000000, 0.000000000000000000, -0.000000000000000000 ) ) ;
#20479=DIRECTION ( 'NONE',  ( 0.000000000000000000, 0.000000000000000000, 1.000000000000000000 ) ) ;
#20490=VERTEX_POINT ( 'NONE', #7044 ) ;
#20492=ORIENTED_EDGE ( 'NONE', *, *, #301, .F. ) ;
#20495=LINE ( 'NONE', #15349, #11987 ) ;
#20496=CIRCLE ( 'NONE', #11459, 10.00000000000000000 ) ;
#20500=DIRECTION ( 'NONE',  ( 1.000000000000000000, 0.000000000000000000, -0.000000000000000000 ) ) ;
#20504=ADVANCED_FACE ( 'NONE', ( #10277 ), #2527, .T. ) ;
#20508=ORIENTED_EDGE ( 'NONE', *, *, #11522, .T. ) ;
#20515=ORIENTED_EDGE ( 'NONE', *, *, #19919, .T. ) ;
#20519=CARTESIAN_POINT ( 'NONE',  ( -11.75209451496117197, 10.00000000000000000, 0.000000000000000000 ) ) ;
#20520=VERTEX_POINT ( 'NONE', #964 ) ;
#20523=ADVANCED_FACE ( 'NONE', ( #4207 ), #8713, .T. ) ;
#20524=CARTESIAN_POINT ( 'NONE',  ( 16.37779268661489596, 0.000000000000000000, 1.000000000000000000 ) ) ;
#20526=DIRECTION ( 'NONE',  ( 1.000000000000000000, 0.000000000000000000, -0.000000000000000000 ) ) ;
#20535=ORIENTED_EDGE ( 'NONE', *, *, #14507, .F. ) ;
#20538=VERTEX_POINT ( 'NONE', #7767 ) ;
#20541=DIRECTION ( 'NONE',  ( 1.000000000000000000, 0.000000000000000000, 0.000000000000000000 ) ) ;
#20544=ADVANCED_FACE ( 'NONE', ( #1179 ), #11110, .T. ) ;
#20551=LINE ( 'NONE', #3172, #14395 ) ;
#20555=ORIENTED_EDGE ( 'NONE', *, *, #9322, .F. ) ;
#20557=CARTESIAN_POINT ( 'NONE',  ( -17.94064177244175795, 0.000000000000000000, 1.000000000000000000 ) ) ;
#20564=EDGE_LOOP ( 'NONE', ( #3082, #14645, #18987, #832 ) ) ;
#20569=ORIENTED_EDGE ( 'NONE', *, *, #13895, .F. ) ;
#20570=CARTESIAN_POINT ( 'NONE',  ( -26.94203811574920593, 0.000000000000000000, 1.000000000000000000 ) ) ;
#20571=CARTESIAN_POINT ( 'NONE',  ( 17.12779268661489596, 16.00000000000000000, 1.000000000000000000 ) ) ;
#20572=CARTESIAN_POINT ( 'NONE',  ( -10.43924542913431175, 10.00000000000000000, 0.000000000000000000 ) ) ;
#20576=CARTESIAN_POINT ( 'NONE',  ( 30.00000000000000000, 10.00000000000000000, 1.000000000000000000 ) ) ;
#20578=DIRECTION ( 'NONE',  ( -0.000000000000000000, 0.000000000000000000, -1.000000000000000000 ) ) ;
#20588=PLANE ( 'NONE',  #10641 ) ;
#20594=PLANE ( 'NONE',  #19004 ) ;
#20602=ORIENTED_EDGE ( 'NONE', *, *, #11091, .F. ) ;
#20613=ORIENTED_EDGE ( 'NONE', *, *, #17937, .T. ) ;
#20616=ADVANCED_FACE ( 'NONE', ( #19173 ), #20438, .T. ) ;
#20617=ORIENTED_EDGE ( 'NONE', *, *, #1, .F. ) ;
#20622=LINE ( 'NONE', #1473, #6390 ) ;
#20631=VERTEX_POINT ( 'NONE', #14756 ) ;
#20641=EDGE_CURVE ( 'NONE', #15727, #1770, #13016, .T. ) ;
#20644=DIRECTION ( 'NONE',  ( 0.000000000000000000, -1.000000000000000000, 0.000000000000000000 ) ) ;
#20648=ORIENTED_EDGE ( 'NONE', *, *, #18360, .T. ) ;
#20655=EDGE_LOOP ( 'NONE', ( #2606, #7304, #9176, #18288 ) ) ;
#20663=LINE ( 'NONE', #14366, #3567 ) ;
#20665=VERTEX_POINT ( 'NONE', #1694 ) ;
#20666=DIRECTION ( 'NONE',  ( 0.000000000000000000, 1.000000000000000000, -0.000000000000000000 ) ) ;
#20676=VECTOR ( 'NONE', #19823, 1000.000000000000114 ) ;
#20680=EDGE_CURVE ( 'NONE', #15361, #3979, #16126, .T. ) ;
#20683=ORIENTED_EDGE ( 'NONE', *, *, #10118, .F. ) ;
#20684=EDGE_CURVE ( 'NONE', #5093, #965, #11412, .T. ) ;
#20686=DIRECTION ( 'NONE',  ( -0.4999999999999949485, 0.8660254037844415942, 0.000000000000000000 ) ) ;
#20687=ORIENTED_EDGE ( 'NONE', *, *, #16821, .F. ) ;
#20692=VECTOR ( 'NONE', #2537, 1000.000000000000000 ) ;
#20695=ADVANCED_FACE ( 'NONE', ( #5139 ), #19678, .T. ) ;
#20697=VECTOR ( 'NONE', #9100, 1000.000000000000000 ) ;
#20707=VECTOR ( 'NONE', #1756, 1000.000000000000000 ) ;
#20712=LINE ( 'NONE', #3331, #18689 ) ;
#20714=VERTEX_POINT ( 'NONE', #11305 ) ;
#20715=DIRECTION ( 'NONE',  ( 0.000000000000000000, -0.000000000000000000, 1.000000000000000000 ) ) ;
#20718=CIRCLE ( 'NONE', #7688, 10.00000000000000000 ) ;
ENDSEC;
END-ISO-10303-21;
